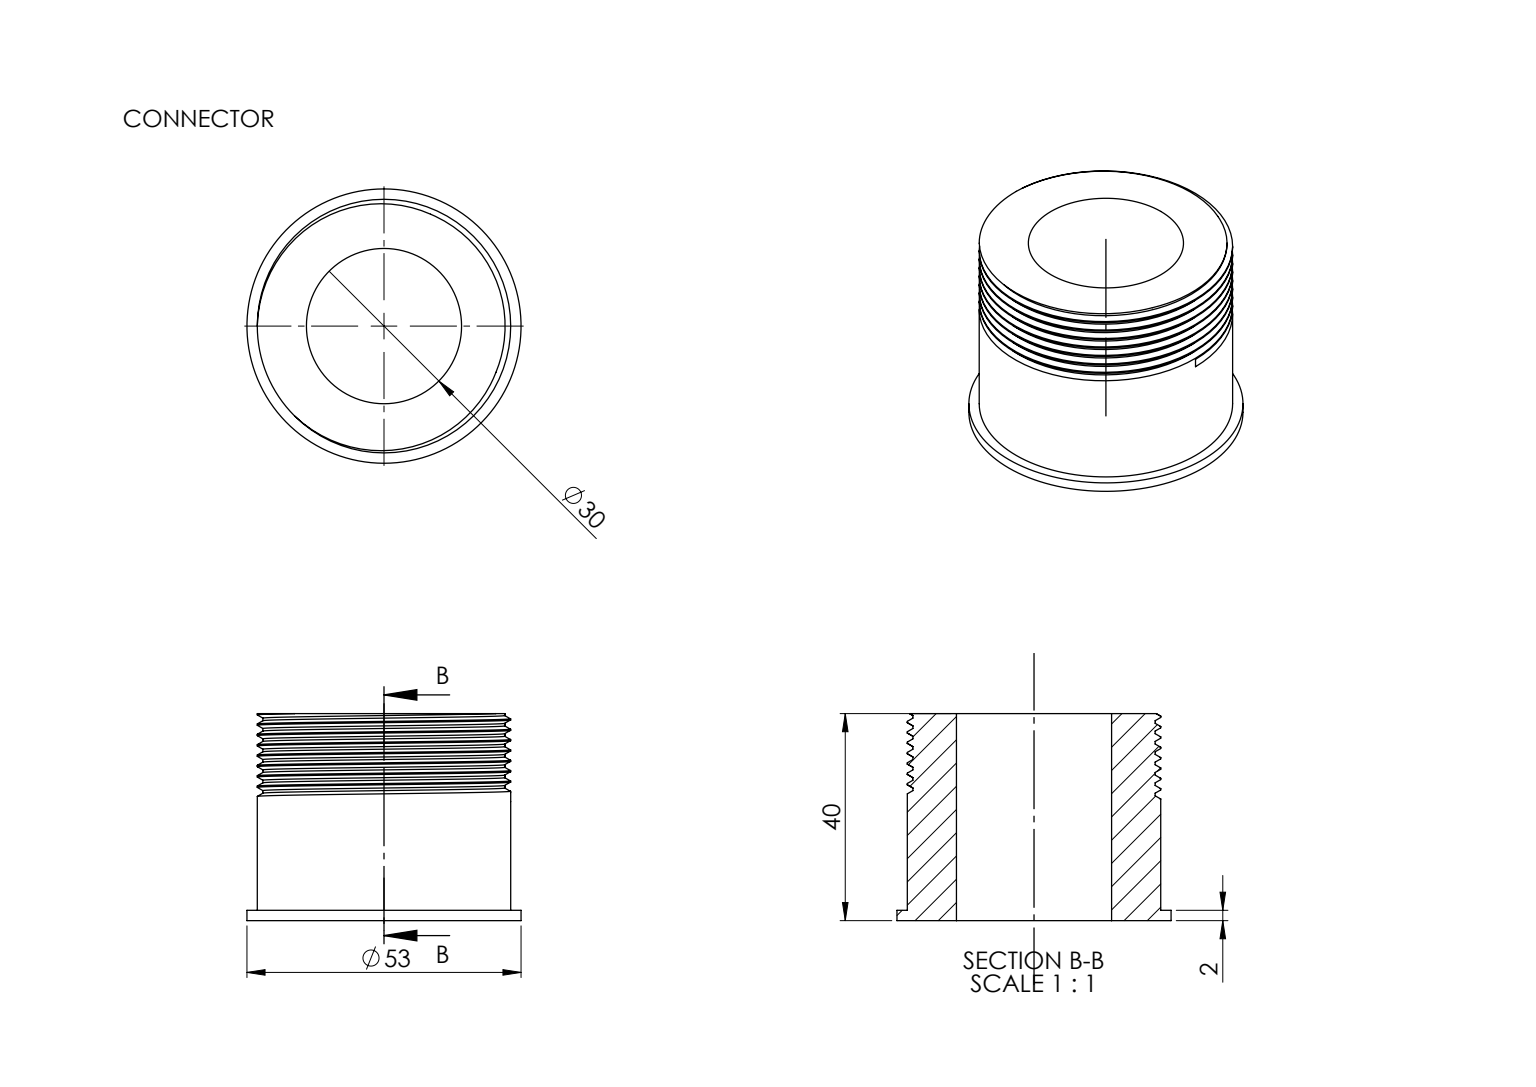
ISO-10303-21;
HEADER;
FILE_DESCRIPTION (('STEP AP214'),
    '1' );
FILE_NAME ('connector.step',
    '2026-10-02T18:08:48',
    ( '' ),
    ( '' ),
    'SwSTEP 2.0',
    'SolidWorks 2026',
    '' );
FILE_SCHEMA (( 'AUTOMOTIVE_DESIGN' ));
ENDSEC;

DATA;
#3=CARTESIAN_POINT ( 'NONE',  ( 7.236395654485760609, 11.52499999726880375, -22.27133577429736633 ) ) ;
#13=CARTESIAN_POINT ( 'NONE',  ( 15.14183272437242067, 5.449999994537614967, 20.84094480462498211 ) ) ;
#22=CARTESIAN_POINT ( 'NONE',  ( 14.47279130897151589, 4.324999997268801799, 19.92008829642072953 ) ) ;
#31=DIRECTION ( 'NONE',  ( 0.000000000000000000, -1.000000000000000000, 0.000000000000000000 ) ) ;
#45=CARTESIAN_POINT ( 'NONE',  ( -14.47279130897151589, 9.324999997268816898, -19.92008829642072598 ) ) ;
#55=EDGE_LOOP ( 'NONE', ( #23841, #28367, #25851, #31674 ) ) ;
#70=CARTESIAN_POINT ( 'NONE',  ( -15.14183272437242600, 17.04999999453762527, 20.84094480462497856 ) ) ;
#86=CARTESIAN_POINT ( 'NONE',  ( -7.236395654485757944, 9.724999997268806595, -22.27133577429736988 ) ) ;
#96=DIRECTION ( 'NONE',  ( 0.000000000000000000, -1.000000000000000000, 0.000000000000000000 ) ) ;
#115=CARTESIAN_POINT ( 'NONE',  ( 0.000000000000000000, 16.99999999999998579, -15.00000000000000000 ) ) ;
#149=CARTESIAN_POINT ( 'NONE',  ( 7.570916362186213000, 8.399999999999991473, -23.30088464923126423 ) ) ;
#161=FACE_OUTER_BOUND ( 'NONE', #7601, .T. ) ;
#173=CARTESIAN_POINT ( 'NONE',  ( -4.523095164977117273E-15, 14.62499999726882649, 24.62258325217400312 ) ) ;
#181=EDGE_CURVE ( 'NONE', #2430, #476, #12819, .T. ) ;
#191=CARTESIAN_POINT ( 'NONE',  ( -7.236395654485763274, 6.024999997268825958, 22.27133577429736633 ) ) ;
#214=CARTESIAN_POINT ( 'NONE',  ( -4.523095164977116484E-15, 12.12499999726881406, 24.62258325217400312 ) ) ;
#242=CARTESIAN_POINT ( 'NONE',  ( 7.236395654485755280, 2.724999997268801266, 22.27133577429736988 ) ) ;
#245=( BOUNDED_CURVE ( )  B_SPLINE_CURVE ( 2, ( #20282, #2248, #31077, #20802, #5337, #28338, #4995 ),
 .UNSPECIFIED., .F., .T. ) 
 B_SPLINE_CURVE_WITH_KNOTS ( ( 3, 2, 2, 3 ),
 ( 0.000000000000000000, 0.01111111111111111154, 0.02222222222222222307, 0.02777777777777777971 ),
 .UNSPECIFIED. ) 
 CURVE ( )  GEOMETRIC_REPRESENTATION_ITEM ( )  RATIONAL_B_SPLINE_CURVE ( ( 1.000000000000000000, 0.9510565162951535312, 1.000000000000000000, 0.9510565162951535312, 1.000000000000000000, 0.9755282581475768211, 0.9755282581475768211 ) ) 
 REPRESENTATION_ITEM ( '' )  );
#257=CARTESIAN_POINT ( 'NONE',  ( -14.47279130897151589, 7.824999997268807128, -19.92008829642072598 ) ) ;
#280=PRODUCT_CONTEXT ( 'NONE', #6136, 'mechanical' ) ;
#294=CARTESIAN_POINT ( 'NONE',  ( 5.270191272235265068, 16.99999999999999645, -22.91526030449972851 ) ) ;
#314=MECHANICAL_DESIGN_GEOMETRIC_PRESENTATION_REPRESENTATION('',(#29900),#24959);
#322=CARTESIAN_POINT ( 'NONE',  ( -7.570916362186215665, 7.399999999999989697, 23.30088464923126423 ) ) ;
#327=CARTESIAN_POINT ( 'NONE',  ( -23.41746824999999887, 1.624999997268811169, -2.867812753649727150E-15 ) ) ;
#328=ADVANCED_FACE ( 'NONE', ( #23862 ), #25917, .T. ) ;
#348=( BOUNDED_CURVE ( )  B_SPLINE_CURVE ( 2, ( #28685, #12736, #2613, #13, #28179, #10501, #4666, #28512, #9994, #20980, #17898, #2090, #20467 ),
 .UNSPECIFIED., .F., .T. ) 
 B_SPLINE_CURVE_WITH_KNOTS ( ( 3, 2, 2, 2, 2, 2, 3 ),
 ( 0.1944444444444444475, 0.2000000000000000111, 0.2111111111111111105, 0.2222222222222222099, 0.2333333333333333370, 0.2444444444444444364, 0.2500000000000000000 ),
 .UNSPECIFIED. ) 
 CURVE ( )  GEOMETRIC_REPRESENTATION_ITEM ( )  RATIONAL_B_SPLINE_CURVE ( ( 0.9755282581475768211, 0.9755282581475768211, 1.000000000000000000, 0.9510565162951535312, 1.000000000000000000, 0.9510565162951535312, 1.000000000000000000, 0.9510565162951535312, 1.000000000000000000, 0.9510565162951535312, 1.000000000000000000, 0.9755282581475767101, 0.9755282581475768211 ) ) 
 REPRESENTATION_ITEM ( '' )  );
#365=CARTESIAN_POINT ( 'NONE',  ( -23.41746825000000243, 7.524999997268816188, -7.608796670333730638 ) ) ;
#375=CARTESIAN_POINT ( 'NONE',  ( 7.236395654485755280, 18.72499999726881370, 22.27133577429736988 ) ) ;
#389=CYLINDRICAL_SURFACE ( 'NONE', #32540, 24.50000000000000000 ) ;
#413=CARTESIAN_POINT ( 'NONE',  ( -18.94512977948576093, 2.324999997268817342, 13.76444248337722698 ) ) ;
#428=CARTESIAN_POINT ( 'NONE',  ( 18.94512977948575738, 14.92499999726881654, 13.76444248337723408 ) ) ;
#430=EDGE_LOOP ( 'NONE', ( #16909, #1055, #4151, #23333 ) ) ;
#441=CARTESIAN_POINT ( 'NONE',  ( -4.223320258572819786E-15, 3.499999999999996891, 24.50000000000000000 ) ) ;
#469=CARTESIAN_POINT ( 'NONE',  ( -24.50000000000000000, 10.74999999453762811, -3.000384657911015469E-15 ) ) ;
#476=VERTEX_POINT ( 'NONE', #13893 ) ;
#492=CARTESIAN_POINT ( 'NONE',  ( -24.50000000000000000, 5.000000000000004441, -3.000384657911015469E-15 ) ) ;
#497=CARTESIAN_POINT ( 'NONE',  ( -23.41746824999999887, 5.624999997268814944, -2.867812753649727150E-15 ) ) ;
#498=CARTESIAN_POINT ( 'NONE',  ( 6.001560367445586717E-15, 3.249999994537631665, 24.50000000000000000 ) ) ;
#505=CYLINDRICAL_SURFACE ( 'NONE', #10621, 24.50000000000000000 ) ;
#515=CARTESIAN_POINT ( 'NONE',  ( -4.523095164977117273E-15, 16.62499999726881583, 24.62258325217400312 ) ) ;
#516=ORIENTED_EDGE ( 'NONE', *, *, #16090, .F. ) ;
#531=CARTESIAN_POINT ( 'NONE',  ( -7.236395654485763274, 8.024999997268828622, 22.27133577429736633 ) ) ;
#539=CARTESIAN_POINT ( 'NONE',  ( 14.47279130897151767, 17.42499999726882365, -19.92008829642072598 ) ) ;
#549=EDGE_CURVE ( 'NONE', #23152, #22342, #16936, .T. ) ;
#554=CARTESIAN_POINT ( 'NONE',  ( 1.507698388325705758E-15, 15.12499999726880873, -24.62258325217400312 ) ) ;
#578=CARTESIAN_POINT ( 'NONE',  ( 24.50000000000000355, 17.84999999453763309, -7.960532557706203605 ) ) ;
#591=CARTESIAN_POINT ( 'NONE',  ( -18.94512977948575738, 11.92499999726881477, -13.76444248337723231 ) ) ;
#594=FACE_OUTER_BOUND ( 'NONE', #26488, .T. ) ;
#609=EDGE_CURVE ( 'NONE', #1393, #3518, #27447, .T. ) ;
#618=EDGE_CURVE ( 'NONE', #4913, #19128, #19343, .T. ) ;
#619=CARTESIAN_POINT ( 'NONE',  ( -19.82091636218621389, 11.19999999999998863, 14.40073868116558842 ) ) ;
#629=CARTESIAN_POINT ( 'NONE',  ( -7.579748464070167083E-14, 12.24999999453762456, -24.50000000000000000 ) ) ;
#658=CARTESIAN_POINT ( 'NONE',  ( 7.570916362186213000, 10.39999999999999325, -23.30088464923126423 ) ) ;
#660=CARTESIAN_POINT ( 'NONE',  ( -15.14183272437241889, 8.449999994537634507, -20.84094480462497856 ) ) ;
#662=CARTESIAN_POINT ( 'NONE',  ( 23.41746824999999887, 10.62499999726881938, 0.000000000000000000 ) ) ;
#666=CARTESIAN_POINT ( 'NONE',  ( 23.41705066890375520, 16.99999999999998934, -0.7769985253002599235 ) ) ;
#683=CARTESIAN_POINT ( 'NONE',  ( 18.94512977948575738, 12.92499999726881654, 13.76444248337723408 ) ) ;
#697=CARTESIAN_POINT ( 'NONE',  ( 7.236395654485755280, 12.22499999726881015, 22.27133577429736988 ) ) ;
#719=CARTESIAN_POINT ( 'NONE',  ( -18.94512977948576093, 15.82499999726880091, 13.76444248337722698 ) ) ;
#744=CARTESIAN_POINT ( 'NONE',  ( -19.82091636218621389, 18.94999999453764161, 14.40073868116558842 ) ) ;
#750=AXIS2_PLACEMENT_3D ( 'NONE', #9964, #23009, #11849 ) ;
#764=CARTESIAN_POINT ( 'NONE',  ( 14.47279130897151767, 15.42499999726879878, -19.92008829642072598 ) ) ;
#795=CARTESIAN_POINT ( 'NONE',  ( -3.331698596277962388, 16.99999999999997868, 23.93330680440991998 ) ) ;
#826=CARTESIAN_POINT ( 'NONE',  ( -24.50000000000000000, 9.000000000000007105, -3.000384657911015469E-15 ) ) ;
#829=CARTESIAN_POINT ( 'NONE',  ( 14.47279130897151767, 12.32499999726880802, 19.92008829642072953 ) ) ;
#844=CARTESIAN_POINT ( 'NONE',  ( -19.82091636218621034, 16.80000000000000782, -14.40073868116559552 ) ) ;
#855=DIRECTION ( 'NONE',  ( 0.000000000000000000, -1.000000000000000000, 0.000000000000000000 ) ) ;
#863=CARTESIAN_POINT ( 'NONE',  ( 18.94512977948575738, 12.42499999726881477, 13.76444248337723408 ) ) ;
#885=CARTESIAN_POINT ( 'NONE',  ( 7.236395654485760609, 13.02499999726880375, -22.27133577429736633 ) ) ;
#890=CARTESIAN_POINT ( 'NONE',  ( -14.47279130897152299, 4.424999997268826313, 19.92008829642072243 ) ) ;
#910=ORIENTED_EDGE ( 'NONE', *, *, #33041, .T. ) ;
#911=CARTESIAN_POINT ( 'NONE',  ( 7.236395654485760609, 9.524999997268828622, -22.27133577429736633 ) ) ;
#926=CARTESIAN_POINT ( 'NONE',  ( -7.236395654485763274, 14.52499999726880553, 22.27133577429736633 ) ) ;
#935=CARTESIAN_POINT ( 'NONE',  ( -3.880418787951137816, 0.5512542815468468582, -24.49999999999999645 ) ) ;
#956=CARTESIAN_POINT ( 'NONE',  ( -6.700584085799521361, 16.99999999999998934, 23.28199799329060582 ) ) ;
#963=CARTESIAN_POINT ( 'NONE',  ( -3.880418787951156023, 10.30125427608447453, -24.49999999999999645 ) ) ;
#975=CARTESIAN_POINT ( 'NONE',  ( 24.50000000000000000, 15.84999999453763664, -7.960532557706203605 ) ) ;
#986=CARTESIAN_POINT ( 'NONE',  ( -24.50000000000000355, 14.89999999999999680, -7.960532557706207157 ) ) ;
#990=CARTESIAN_POINT ( 'NONE',  ( -7.236395654485763274, 10.02499999726880198, 22.27133577429736633 ) ) ;
#991=CARTESIAN_POINT ( 'NONE',  ( -1.756012107511856980E-14, 4.499999999999997335, -24.50000000000000000 ) ) ;
#994=CARTESIAN_POINT ( 'NONE',  ( 19.05376897654620194, 16.99999999999997868, -13.63518129362208953 ) ) ;
#1023=CARTESIAN_POINT ( 'NONE',  ( 18.94512977948576093, 12.82499999726882578, -13.76444248337722875 ) ) ;
#1049=CARTESIAN_POINT ( 'NONE',  ( -23.41746825000000243, 4.224999997268803931, 7.608796670333725309 ) ) ;
#1055=ORIENTED_EDGE ( 'NONE', *, *, #4319, .F. ) ;
#1072=CARTESIAN_POINT ( 'NONE',  ( -14.47279130897151589, 7.824999997268807128, -19.92008829642072598 ) ) ;
#1082=CARTESIAN_POINT ( 'NONE',  ( -7.579748464070165821E-14, 16.50000000000000355, -24.50000000000000000 ) ) ;
#1087=CARTESIAN_POINT ( 'NONE',  ( 23.41746825000000243, 17.22499999726880304, -7.608796670333727974 ) ) ;
#1095=CARTESIAN_POINT ( 'NONE',  ( -24.50000000000000000, 0.9000000000000005773, -7.960532557706207157 ) ) ;
#1096=EDGE_LOOP ( 'NONE', ( #14624, #31167 ) ) ;
#1109=CARTESIAN_POINT ( 'NONE',  ( -15.14183272437242067, 16.44999999453761674, -20.84094480462497856 ) ) ;
#1110=CARTESIAN_POINT ( 'NONE',  ( 7.313012447739250820E-14, 15.50000000000000178, 24.50000000000000000 ) ) ;
#1116=CARTESIAN_POINT ( 'NONE',  ( 20.86390607985937606, 16.99999999999997868, 10.74782858706267952 ) ) ;
#1153=CARTESIAN_POINT ( 'NONE',  ( 24.50000000000000000, 12.00000000000001066, 0.000000000000000000 ) ) ;
#1157=CARTESIAN_POINT ( 'NONE',  ( -14.47279130897152299, 11.92499999726882187, 19.92008829642072243 ) ) ;
#1159=CARTESIAN_POINT ( 'NONE',  ( 19.82091636218621389, 3.949999994537628289, -14.40073868116559197 ) ) ;
#1193=CARTESIAN_POINT ( 'NONE',  ( -4.523095164977116484E-15, 10.12499999726881938, 24.62258325217400312 ) ) ;
#1199=ORIENTED_EDGE ( 'NONE', *, *, #16507, .F. ) ;
#1229=CARTESIAN_POINT ( 'NONE',  ( -1.756012107511856980E-14, 4.499999999999997335, -24.50000000000000000 ) ) ;
#1232=( BOUNDED_CURVE ( )  B_SPLINE_CURVE ( 2, ( #19854, #17980, #28430, #1483, #30308, #11957, #32875, #6807, #9374, #17286, #27749, #14711, #441 ),
 .UNSPECIFIED., .F., .T. ) 
 B_SPLINE_CURVE_WITH_KNOTS ( ( 3, 2, 2, 2, 2, 2, 3 ),
 ( 0.1388888888888888951, 0.1444444444444444309, 0.1555555555555555580, 0.1666666666666666574, 0.1777777777777777846, 0.1888888888888888840, 0.1944444444444444475 ),
 .UNSPECIFIED. ) 
 CURVE ( )  GEOMETRIC_REPRESENTATION_ITEM ( )  RATIONAL_B_SPLINE_CURVE ( ( 0.9755282581475768211, 0.9755282581475768211, 1.000000000000000000, 0.9510565162951535312, 1.000000000000000000, 0.9510565162951535312, 1.000000000000000000, 0.9510565162951535312, 1.000000000000000000, 0.9510565162951535312, 1.000000000000000000, 0.9755282581475768211, 0.9755282581475768211 ) ) 
 REPRESENTATION_ITEM ( '' )  );
#1241=CARTESIAN_POINT ( 'NONE',  ( -23.41746825000000598, 4.224999997268803931, 7.608796670333726198 ) ) ;
#1255=CARTESIAN_POINT ( 'NONE',  ( -4.523095164977116484E-15, 18.62499999726881583, 24.62258325217400312 ) ) ;
#1263=ORIENTED_EDGE ( 'NONE', *, *, #19113, .T. ) ;
#1281=CARTESIAN_POINT ( 'NONE',  ( 19.82091636218621034, 9.549999994537621717, 14.40073868116559730 ) ) ;
#1295=CARTESIAN_POINT ( 'NONE',  ( 23.41746825000000243, 3.024999997268812635, 7.608796670333735079 ) ) ;
#1324=CARTESIAN_POINT ( 'NONE',  ( 19.82091636218621034, 9.800000000000002487, 14.40073868116559730 ) ) ;
#1329=CARTESIAN_POINT ( 'NONE',  ( 23.41746824999999887, 12.52499999726880375, 7.608796670333735079 ) ) ;
#1334=CARTESIAN_POINT ( 'NONE',  ( -7.570916362186215665, 5.149999994537635573, 23.30088464923126423 ) ) ;
#1335=DIRECTION ( 'NONE',  ( -0.8660254037844399289, -0.4999999999999977240, 0.000000000000000000 ) ) ;
#1366=CARTESIAN_POINT ( 'NONE',  ( 23.41746825000000243, 10.72499999726880127, -7.608796670333727974 ) ) ;
#1373=EDGE_CURVE ( 'NONE', #11531, #13996, #14522, .T. ) ;
#1376=AXIS2_PLACEMENT_3D ( 'NONE', #6186, #27460, #21818 ) ;
#1378=CARTESIAN_POINT ( 'NONE',  ( 3.000384657911015469E-15, 16.99999999999998579, 24.50000000000000000 ) ) ;
#1393=VERTEX_POINT ( 'NONE', #7954 ) ;
#1409=SURFACE_SIDE_STYLE ('',( #16544 ) ) ;
#1416=CARTESIAN_POINT ( 'NONE',  ( 23.41746825000000243, 9.024999997268826846, 7.608796670333735079 ) ) ;
#1427=CARTESIAN_POINT ( 'NONE',  ( 7.570916362186207671, 7.349999994537615322, 23.30088464923126779 ) ) ;
#1429=CARTESIAN_POINT ( 'NONE',  ( 23.41746825000000243, 4.724999997268818142, -7.608796670333727974 ) ) ;
#1454=CARTESIAN_POINT ( 'NONE',  ( -19.82091636218621034, 4.549999994537618164, -14.40073868116559552 ) ) ;
#1463=ADVANCED_FACE ( 'NONE', ( #2982 ), #389, .T. ) ;
#1471=CARTESIAN_POINT ( 'NONE',  ( 14.47279130897151589, 2.824999997268819119, 19.92008829642072953 ) ) ;
#1483=CARTESIAN_POINT ( 'NONE',  ( -15.14183272437242067, 2.700000000000001954, -20.84094480462497856 ) ) ;
#1497=CARTESIAN_POINT ( 'NONE',  ( -15.14183272437241889, 16.69999999999999574, -20.84094480462497856 ) ) ;
#1501=CARTESIAN_POINT ( 'NONE',  ( 23.41746824999999887, 16.62499999726882294, 0.000000000000000000 ) ) ;
#1536=CARTESIAN_POINT ( 'NONE',  ( 14.47279130897151767, 14.92499999726881299, -19.92008829642072598 ) ) ;
#1558=CARTESIAN_POINT ( 'NONE',  ( 23.41746824999999887, 3.124999997268812280, 0.000000000000000000 ) ) ;
#1575=DIRECTION ( 'NONE',  ( 0.000000000000000000, -1.000000000000000000, 0.000000000000000000 ) ) ;
#1582=CARTESIAN_POINT ( 'NONE',  ( -18.94512977948576093, 4.324999997268818674, 13.76444248337722698 ) ) ;
#1594=CARTESIAN_POINT ( 'NONE',  ( -14.47279130897152122, 5.924999997268808549, 19.92008829642072243 ) ) ;
#1618=CARTESIAN_POINT ( 'NONE',  ( 1.555960095263670572E-15, 14.24999999453762278, -24.50000000000000000 ) ) ;
#1620=CARTESIAN_POINT ( 'NONE',  ( 7.570916362186213000, 4.149999994537633796, -23.30088464923126423 ) ) ;
#1634=CARTESIAN_POINT ( 'NONE',  ( -14.47279130897152122, 2.424999997268802332, 19.92008829642072243 ) ) ;
#1648=CARTESIAN_POINT ( 'NONE',  ( 1.555960095263670572E-15, 8.249999994537619230, -24.50000000000000000 ) ) ;
#1669=CARTESIAN_POINT ( 'NONE',  ( 18.94512977948576093, 14.82499999726880091, -13.76444248337722875 ) ) ;
#1673=CARTESIAN_POINT ( 'NONE',  ( -4.223320258572819786E-15, 5.249999994537629888, 24.50000000000000000 ) ) ;
#1704=CARTESIAN_POINT ( 'NONE',  ( 24.50000000000000355, 0.09999999999999684142, -7.960532557706203605 ) ) ;
#1728=CARTESIAN_POINT ( 'NONE',  ( -7.236395654485757944, 5.724999997268803931, -22.27133577429736988 ) ) ;
#1748=CARTESIAN_POINT ( 'NONE',  ( 19.82091636218621389, 8.200000000000013500, -14.40073868116559197 ) ) ;
#1751=ORIENTED_EDGE ( 'NONE', *, *, #28129, .T. ) ;
#1752=CARTESIAN_POINT ( 'NONE',  ( 23.41746824999999887, 13.12499999726882116, 0.000000000000000000 ) ) ;
#1753=CARTESIAN_POINT ( 'NONE',  ( 23.41746824999999887, 0.6249999972688102812, 0.000000000000000000 ) ) ;
#1765=CARTESIAN_POINT ( 'NONE',  ( 18.94512977948576093, 0.8249999972688160099, -13.76444248337722875 ) ) ;
#1793=CARTESIAN_POINT ( 'NONE',  ( -4.732186688966233175E-15, 7.249999994537616566, 25.76082449383753925 ) ) ;
#1809=CARTESIAN_POINT ( 'NONE',  ( -7.236395654485757944, 3.724999997268802154, -22.27133577429736988 ) ) ;
#1844=FACE_OUTER_BOUND ( 'NONE', #14245, .T. ) ;
#1875=CARTESIAN_POINT ( 'NONE',  ( 24.50000000000000000, 13.64999999453761781, 7.960532557706212486 ) ) ;
#1880=CARTESIAN_POINT ( 'NONE',  ( -15.14183272437241889, 0.7000000000000070610, -20.84094480462497856 ) ) ;
#1882=DIRECTION ( 'NONE',  ( 0.000000000000000000, -0.000000000000000000, -1.000000000000000000 ) ) ;
#1907=CARTESIAN_POINT ( 'NONE',  ( 14.47279130897151767, 8.824999997268804464, 19.92008829642072953 ) ) ;
#1927=CARTESIAN_POINT ( 'NONE',  ( 7.570916362186213000, 8.399999999999991473, -23.30088464923126423 ) ) ;
#1931=CARTESIAN_POINT ( 'NONE',  ( 18.94512977948576093, 15.32499999726880091, -13.76444248337722875 ) ) ;
#1932=CARTESIAN_POINT ( 'NONE',  ( 14.47279130897151944, 0.9249999972688209837, -19.92008829642072598 ) ) ;
#1947=CARTESIAN_POINT ( 'NONE',  ( -23.41746825000000243, 3.524999997268826402, -7.608796670333730638 ) ) ;
#1949=STYLED_ITEM ( 'NONE', ( #25225 ), #13626 ) ;
#1952=( BOUNDED_CURVE ( )  B_SPLINE_CURVE ( 2, ( #2358, #18503, #16757, #1109, #19331, #11594, #27216, #6281, #3378, #3709, #14179 ),
 .UNSPECIFIED., .F., .T. ) 
 B_SPLINE_CURVE_WITH_KNOTS ( ( 3, 2, 2, 2, 2, 3 ),
 ( 0.8055555555555555802, 0.8111111111111111160, 0.8222222222222221877, 0.8333333333333333703, 0.8444444444444444420, 0.8472738309268738055 ),
 .UNSPECIFIED. ) 
 CURVE ( )  GEOMETRIC_REPRESENTATION_ITEM ( )  RATIONAL_B_SPLINE_CURVE ( ( 0.9755282581475768211, 0.9755282581475768211, 1.000000000000000000, 0.9510565162951535312, 1.000000000000000000, 0.9510565162951535312, 1.000000000000000000, 0.9510565162951535312, 1.000000000000000000, 0.9875367971922254240, 0.9814209735438276239 ) ) 
 REPRESENTATION_ITEM ( '' )  );
#1961=VECTOR ( 'NONE', #29560, 1000.000000000000000 ) ;
#1974=CARTESIAN_POINT ( 'NONE',  ( 15.14183272437241889, 15.44999999453761852, 20.84094480462498211 ) ) ;
#1987=CARTESIAN_POINT ( 'NONE',  ( -14.47279130897151589, 1.824999997268821339, -19.92008829642072598 ) ) ;
#1993=ORIENTED_EDGE ( 'NONE', *, *, #6515, .F. ) ;
#2021=CARTESIAN_POINT ( 'NONE',  ( 23.41746824999999887, 14.62499999726882294, 0.000000000000000000 ) ) ;
#2022=VECTOR ( 'NONE', #3479, 1000.000000000000000 ) ;
#2026=CARTESIAN_POINT ( 'NONE',  ( -24.50000000000000711, 4.849999994537633974, 7.960532557706201828 ) ) ;
#2038=ORIENTED_EDGE ( 'NONE', *, *, #18277, .T. ) ;
#2056=CARTESIAN_POINT ( 'NONE',  ( 23.41746825000000243, 16.72499999726881725, -7.608796670333727974 ) ) ;
#2062=ORIENTED_EDGE ( 'NONE', *, *, #16915, .F. ) ;
#2071=CARTESIAN_POINT ( 'NONE',  ( 7.570916362186207671, 5.599999999999994316, 23.30088464923126779 ) ) ;
#2075=CARTESIAN_POINT ( 'NONE',  ( 19.82091636218621034, 7.549999994537620829, 14.40073868116559730 ) ) ;
#2082=CARTESIAN_POINT ( 'NONE',  ( -23.41746824999999887, 8.024999997268800200, -7.608796670333730638 ) ) ;
#2090=CARTESIAN_POINT ( 'NONE',  ( 3.880418787951132042, 6.198745712990783474, -24.50000000000000355 ) ) ;
#2098=CARTESIAN_POINT ( 'NONE',  ( -18.94512977948575738, 1.424999997268805441, -13.76444248337723231 ) ) ;
#2107=CARTESIAN_POINT ( 'NONE',  ( 14.47279130897151589, 14.82499999726881690, 19.92008829642072953 ) ) ;
#2108=CARTESIAN_POINT ( 'NONE',  ( 18.94512977948575738, 4.424999997268807661, 13.76444248337723408 ) ) ;
#2120=CARTESIAN_POINT ( 'NONE',  ( -23.41746825000000243, 9.524999997268810858, -7.608796670333730638 ) ) ;
#2143=CARTESIAN_POINT ( 'NONE',  ( 19.82091636218621034, 15.54999999453762705, 14.40073868116559730 ) ) ;
#2157=CARTESIAN_POINT ( 'NONE',  ( 14.47279130897151589, 10.82499999726882756, 19.92008829642072953 ) ) ;
#2184=CARTESIAN_POINT ( 'NONE',  ( -24.50000000000000000, 16.99999999999998579, -3.000384657911015469E-15 ) ) ;
#2189=CARTESIAN_POINT ( 'NONE',  ( -7.236395654485763274, 16.02499999726880731, 22.27133577429736633 ) ) ;
#2206=DIRECTION ( 'NONE',  ( 0.000000000000000000, -1.000000000000000000, 0.000000000000000000 ) ) ;
#2220=( NAMED_UNIT ( * ) PLANE_ANGLE_UNIT ( ) SI_UNIT ( $, .RADIAN. ) );
#2224=CARTESIAN_POINT ( 'NONE',  ( 23.41746825000000243, 16.52499999726882152, 7.608796670333735079 ) ) ;
#2248=CARTESIAN_POINT ( 'NONE',  ( 24.50000000000000000, 0.09999999999999682754, -7.960532557706203605 ) ) ;
#2253=CARTESIAN_POINT ( 'NONE',  ( 14.47279130897151944, 7.424999997268819207, -19.92008829642072598 ) ) ;
#2271=CARTESIAN_POINT ( 'NONE',  ( 18.94512977948576093, 0.8249999972688160099, -13.76444248337722875 ) ) ;
#2280=CARTESIAN_POINT ( 'NONE',  ( 23.41746824999999887, 11.12499999726881938, 0.000000000000000000 ) ) ;
#2281=CARTESIAN_POINT ( 'NONE',  ( 18.94512977948576093, 4.824999997268819563, -13.76444248337722875 ) ) ;
#2296=CARTESIAN_POINT ( 'NONE',  ( -14.47279130897151589, 11.32499999726881157, -19.92008829642072598 ) ) ;
#2298=ORIENTED_EDGE ( 'NONE', *, *, #30160, .T. ) ;
#2319=CARTESIAN_POINT ( 'NONE',  ( -15.14183272437242600, 13.04999999453763770, 20.84094480462497856 ) ) ;
#2333=AXIS2_PLACEMENT_3D ( 'NONE', #21565, #16419, #19157 ) ;
#2334=CARTESIAN_POINT ( 'NONE',  ( -7.236395654485757944, 5.724999997268803931, -22.27133577429736988 ) ) ;
#2339=ORIENTED_EDGE ( 'NONE', *, *, #18402, .F. ) ;
#2358=CARTESIAN_POINT ( 'NONE',  ( 1.555960095263670572E-15, 16.24999999453762101, -24.50000000000000000 ) ) ;
#2368=B_SPLINE_CURVE_WITH_KNOTS ( 'NONE', 3,
 ( #13729, #11643, #22127, #32240, #9070, #31901, #19550, #16976, #29653, #32403, #8396, #16642, #994, #6333, #18883, #11479, #13569, #5833, #16471, #3259, #24196, #29491, #666, #5995, #12148, #30852, #4260, #25546, #32737, #25195, #27947, #25025 ),
 .UNSPECIFIED., .F., .F.,
 ( 4, 2, 2, 2, 2, 2, 2, 2, 2, 2, 2, 2, 2, 2, 2, 4 ),
 ( 0.000000000000000000, 0.002298871809599534188, 0.004597743619199068377, 0.006896615428798602565, 0.009195487238398136753, 0.01149435904799767094, 0.01379323085759720513, 0.01609210266719673932, 0.01839097447679627351, 0.02298871809599534188, 0.02528758990559487607, 0.02758646171519441026, 0.02988533352479394445, 0.03218420533439347864, 0.03448307714399301283, 0.03678194895359254701 ),
 .UNSPECIFIED. ) ;
#2396=EDGE_CURVE ( 'NONE', #3518, #19128, #27625, .T. ) ;
#2405=CARTESIAN_POINT ( 'NONE',  ( 15.14183272437241889, 5.699999999999993960, 20.84094480462498211 ) ) ;
#2411=VECTOR ( 'NONE', #14860, 1000.000000000000000 ) ;
#2417=PLANE ( 'NONE',  #7272 ) ;
#2429=CARTESIAN_POINT ( 'NONE',  ( 23.41746824999999887, 9.024999997268826846, 7.608796670333735079 ) ) ;
#2430=VERTEX_POINT ( 'NONE', #11664 ) ;
#2438=FACE_OUTER_BOUND ( 'NONE', #21729, .T. ) ;
#2456=CARTESIAN_POINT ( 'NONE',  ( -23.41746825000000598, 12.22499999726881370, 7.608796670333726198 ) ) ;
#2457=CARTESIAN_POINT ( 'NONE',  ( 14.47279130897151944, 2.924999997268816099, -19.92008829642072598 ) ) ;
#2469=CARTESIAN_POINT ( 'NONE',  ( 7.236395654485760609, 7.024999997268826846, -22.27133577429736633 ) ) ;
#2471=DIRECTION ( 'NONE',  ( 0.000000000000000000, 0.000000000000000000, -1.000000000000000000 ) ) ;
#2494=CARTESIAN_POINT ( 'NONE',  ( 7.570916362186213000, 14.14999999453761603, -23.30088464923126423 ) ) ;
#2510=CARTESIAN_POINT ( 'NONE',  ( -18.94512977948575738, 5.924999997268809437, -13.76444248337723231 ) ) ;
#2519=ORIENTED_EDGE ( 'NONE', *, *, #7482, .F. ) ;
#2521=CARTESIAN_POINT ( 'NONE',  ( 3.880418787951102289, 10.44874571845314470, -24.50000000000000711 ) ) ;
#2529=CARTESIAN_POINT ( 'NONE',  ( -19.82091636218621034, 4.799999999999998934, -14.40073868116559552 ) ) ;
#2542=AXIS2_PLACEMENT_3D ( 'NONE', #19089, #31, #24235 ) ;
#2581=CARTESIAN_POINT ( 'NONE',  ( -24.50000000000000355, 2.899999999999995470, -7.960532557706207157 ) ) ;
#2586=DIRECTION ( 'NONE',  ( 0.000000000000000000, -1.000000000000000000, 0.000000000000000000 ) ) ;
#2590=LINE ( 'NONE', #28030, #25348 ) ;
#2605=CARTESIAN_POINT ( 'NONE',  ( -14.47279130897152299, 12.42499999726880588, 19.92008829642072243 ) ) ;
#2613=CARTESIAN_POINT ( 'NONE',  ( 7.570916362186207671, 5.349999994537641079, 23.30088464923126779 ) ) ;
#2621=CARTESIAN_POINT ( 'NONE',  ( -18.94512977948576093, 5.824999997268820451, 13.76444248337722698 ) ) ;
#2643=CARTESIAN_POINT ( 'NONE',  ( -14.47279130897152122, 9.924999997268825425, 19.92008829642072243 ) ) ;
#2658=CARTESIAN_POINT ( 'NONE',  ( -19.82091636218621034, 6.549999994537619941, -14.40073868116559552 ) ) ;
#2670=CARTESIAN_POINT ( 'NONE',  ( -7.570916362186210335, 10.34999999453761710, -23.30088464923126779 ) ) ;
#2673=( BOUNDED_SURFACE ( )  B_SPLINE_SURFACE ( 1, 2, ( 
 ( #20020, #12111, #9194, #25331, #15043, #33034, #9887, #1987, #19679, #24988, #20364, #27566, #12462, #1634, #22932, #9712, #33388, #1471, #7134, #1295, #25157, #4393, #30812, #22583, #7305, #30125, #1809, #11777, #6795, #6628, #22257, #9538, #17789, #17107, #4053, #11946, #22415, #6965, #32863, #9360, #12285, #22759, #19841, #33210, #12977, #15388, #2334, #18311, #2510, #18478, #23279, #2685, #10574, #33565, #4907, #31664, #10403, #28922, #28583, #8159, #33914, #20882, #7994, #13144, #21221, #31331, #26190, #257, #7823, #28757, #5253, #18649, #29087, #5422, #31501, #15735, #10063, #15902, #18139, #12807, #10239, #23617, #28418, #21052, #15213, #13318, #86, #17968, #23452, #26357, #31161, #2847, #25676, #10742, #25844, #23791, #5080, #2157, #26018, #12631, #23101, #20543, #30988, #7488, #33744, #20720, #15566, #7653, #591, #29425, #22049, #5927, #16404, #18813, #29256, #6256, #3683, #29582, #5759, #8824, #16735, #13824, #19309, #26528, #29751, #27192, #18980, #13988, #3021, #24293, #3354, #24450, #13492, #11245, #926, #19475, #8493, #8660, #428, #5591, #24125, #16073, #21722, #764, #32496, #26859, #14156, #10913, #32167, #6085, #26694, #23957, #11405, #16239, #19144, #24613, #16567, #27022, #3517, #21882, #32332, #1087, #11569, #8995, #11082, #21385, #31830, #8323, #3190, #13661, #31997, #21551, #33171, #4525, #27526, #1255, #9675, #17067, #4015, #27871, #14489 ),
 ( #25295, #9499, #1765, #17409, #30426, #24947, #6925, #4353, #12072, #14829, #22723, #12246, #14322, #25119, #17236, #3847, #19980, #20155, #4187, #15001, #30600, #24777, #30084, #25470, #32663, #7095, #6757, #17579, #28039, #1947, #19641, #12423, #33350, #9318, #32991, #22893, #22379, #9848, #11736, #29925, #6427, #1429, #22216, #16900, #19805, #27362, #9158, #6590, #11907, #32827, #30253, #27696, #14659, #1594, #22542, #31288, #13106, #4870, #25977, #23064, #28884, #17931, #4696, #10027, #2469, #12935, #15350, #7446, #31122, #5382, #20682, #25641, #12593, #18268, #23411, #33701, #10202, #10365, #18440, #33524, #7265, #30775, #18095, #23579, #10533, #20843, #15861, #45, #33872, #2120, #15524, #28381, #7782, #2643, #17751, #28716, #7615, #25804, #28542, #21010, #5212, #31460, #20325, #20501, #26147, #15695, #7953, #2296, #12768, #26317, #2806, #13273, #30949, #23748, #23242, #214, #28210, #15176, #5039, #24086, #16200, #18941, #11367, #11205, #885, #10700, #10873, #16523, #32124, #24248, #26654, #5722, #21843, #13621, #3149, #21348, #13946, #19265, #8280, #16031, #24409, #31789, #18772, #8620, #29216, #554, #11040, #32288, #29386, #21508, #8781, #6042, #719, #26975, #19102, #21676, #31957, #29540, #3475, #26818, #29707, #6210, #16691, #29047, #5886, #8450, #18608, #27148, #3641, #16363, #14115, #24573, #5550, #3314, #21181, #13449, #31623, #13780, #8121, #26486, #2981 ) ),
 .UNSPECIFIED., .F., .F., .T. ) 
 B_SPLINE_SURFACE_WITH_KNOTS ( ( 2, 2 ),
 ( 3, 2, 2, 2, 2, 2, 2, 2, 2, 2, 2, 2, 2, 2, 2, 2, 2, 2, 2, 2, 2, 2, 2, 2, 2, 2, 2, 2, 2, 2, 2, 2, 2, 2, 2, 2, 2, 2, 2, 2, 2, 2, 2, 2, 2, 2, 2, 2, 2, 2, 2, 2, 2, 2, 2, 2, 2, 2, 2, 2, 2, 2, 2, 2, 2, 2, 2, 2, 2, 2, 2, 2, 2, 2, 2, 2, 2, 2, 2, 2, 2, 2, 2, 2, 2, 2, 2, 2, 2, 2, 3 ),
 ( 0.000000000000000000, 1.000000000000000000 ),
 ( 0.000000000000000000, 0.01111111111111111154, 0.02222222222222222307, 0.03333333333333333287, 0.04444444444444444614, 0.05555555555555555247, 0.06666666666666666574, 0.07777777777777777901, 0.08888888888888889228, 0.1000000000000000056, 0.1111111111111111049, 0.1222222222222222182, 0.1333333333333333315, 0.1444444444444444309, 0.1555555555555555580, 0.1666666666666666574, 0.1777777777777777846, 0.1888888888888888840, 0.2000000000000000111, 0.2111111111111111105, 0.2222222222222222099, 0.2333333333333333370, 0.2444444444444444364, 0.2555555555555555358, 0.2666666666666666630, 0.2777777777777777901, 0.2888888888888888618, 0.2999999999999999889, 0.3111111111111111160, 0.3222222222222222432, 0.3333333333333333148, 0.3444444444444444420, 0.3555555555555555691, 0.3666666666666666408, 0.3777777777777777679, 0.3888888888888888951, 0.4000000000000000222, 0.4111111111111110938, 0.4222222222222222210, 0.4333333333333333481, 0.4444444444444444198, 0.4555555555555555469, 0.4666666666666666741, 0.4777777777777778012, 0.4888888888888888729, 0.5000000000000000000, 0.5111111111111110716, 0.5222222222222222543, 0.5333333333333333259, 0.5444444444444443976, 0.5555555555555555802, 0.5666666666666666519, 0.5777777777777777235, 0.5888888888888889062, 0.5999999999999999778, 0.6111111111111111605, 0.6222222222222222321, 0.6333333333333333037, 0.6444444444444444864, 0.6555555555555555580, 0.6666666666666666297, 0.6777777777777778123, 0.6888888888888888840, 0.6999999999999999556, 0.7111111111111111382, 0.7222222222222222099, 0.7333333333333332815, 0.7444444444444444642, 0.7555555555555555358, 0.7666666666666667185, 0.7777777777777777901, 0.7888888888888888618, 0.8000000000000000444, 0.8111111111111111160, 0.8222222222222221877, 0.8333333333333333703, 0.8444444444444444420, 0.8555555555555555136, 0.8666666666666666963, 0.8777777777777777679, 0.8888888888888888395, 0.9000000000000000222, 0.9111111111111110938, 0.9222222222222222765, 0.9333333333333333481, 0.9444444444444444198, 0.9555555555555556024, 0.9666666666666666741, 0.9777777777777777457, 0.9888888888888889284, 1.000000000000000000 ),
 .UNSPECIFIED. ) 
 GEOMETRIC_REPRESENTATION_ITEM ( )  RATIONAL_B_SPLINE_SURFACE ( (
 ( 1.000000000000000000, 0.9510565162951535312, 1.000000000000000000, 0.9510565162951535312, 1.000000000000000000, 0.9510565162951535312, 1.000000000000000000, 0.9510565162951535312, 1.000000000000000000, 0.9510565162951535312, 1.000000000000000000, 0.9510565162951535312, 1.000000000000000000, 0.9510565162951535312, 1.000000000000000000, 0.9510565162951535312, 1.000000000000000000, 0.9510565162951535312, 1.000000000000000000, 0.9510565162951535312, 1.000000000000000000, 0.9510565162951535312, 1.000000000000000000, 0.9510565162951535312, 1.000000000000000000, 0.9510565162951535312, 1.000000000000000000, 0.9510565162951535312, 1.000000000000000000, 0.9510565162951535312, 1.000000000000000000, 0.9510565162951535312, 1.000000000000000000, 0.9510565162951535312, 1.000000000000000000, 0.9510565162951535312, 1.000000000000000000, 0.9510565162951535312, 1.000000000000000000, 0.9510565162951535312, 1.000000000000000000, 0.9510565162951535312, 1.000000000000000000, 0.9510565162951535312, 1.000000000000000000, 0.9510565162951535312, 1.000000000000000000, 0.9510565162951535312, 1.000000000000000000, 0.9510565162951535312, 1.000000000000000000, 0.9510565162951535312, 1.000000000000000000, 0.9510565162951535312, 1.000000000000000000, 0.9510565162951535312, 1.000000000000000000, 0.9510565162951535312, 1.000000000000000000, 0.9510565162951535312, 1.000000000000000000, 0.9510565162951535312, 1.000000000000000000, 0.9510565162951535312, 1.000000000000000000, 0.9510565162951535312, 1.000000000000000000, 0.9510565162951535312, 1.000000000000000000, 0.9510565162951535312, 1.000000000000000000, 0.9510565162951535312, 1.000000000000000000, 0.9510565162951535312, 1.000000000000000000, 0.9510565162951535312, 1.000000000000000000, 0.9510565162951535312, 1.000000000000000000, 0.9510565162951535312, 1.000000000000000000, 0.9510565162951535312, 1.000000000000000000, 0.9510565162951535312, 1.000000000000000000, 0.9510565162951535312, 1.000000000000000000, 0.9510565162951535312, 1.000000000000000000, 0.9510565162951535312, 1.000000000000000000, 0.9510565162951535312, 1.000000000000000000, 0.9510565162951535312, 1.000000000000000000, 0.9510565162951535312, 1.000000000000000000, 0.9510565162951535312, 1.000000000000000000, 0.9510565162951535312, 1.000000000000000000, 0.9510565162951535312, 1.000000000000000000, 0.9510565162951535312, 1.000000000000000000, 0.9510565162951535312, 1.000000000000000000, 0.9510565162951535312, 1.000000000000000000, 0.9510565162951535312, 1.000000000000000000, 0.9510565162951535312, 1.000000000000000000, 0.9510565162951535312, 1.000000000000000000, 0.9510565162951535312, 1.000000000000000000, 0.9510565162951535312, 1.000000000000000000, 0.9510565162951535312, 1.000000000000000000, 0.9510565162951535312, 1.000000000000000000, 0.9510565162951535312, 1.000000000000000000, 0.9510565162951535312, 1.000000000000000000, 0.9510565162951535312, 1.000000000000000000, 0.9510565162951535312, 1.000000000000000000, 0.9510565162951535312, 1.000000000000000000, 0.9510565162951535312, 1.000000000000000000, 0.9510565162951535312, 1.000000000000000000, 0.9510565162951535312, 1.000000000000000000, 0.9510565162951535312, 1.000000000000000000, 0.9510565162951535312, 1.000000000000000000, 0.9510565162951535312, 1.000000000000000000, 0.9510565162951535312, 1.000000000000000000, 0.9510565162951535312, 1.000000000000000000, 0.9510565162951535312, 1.000000000000000000, 0.9510565162951535312, 1.000000000000000000, 0.9510565162951535312, 1.000000000000000000, 0.9510565162951535312, 1.000000000000000000, 0.9510565162951535312, 1.000000000000000000, 0.9510565162951535312, 1.000000000000000000, 0.9510565162951535312, 1.000000000000000000, 0.9510565162951535312, 1.000000000000000000, 0.9510565162951535312, 1.000000000000000000, 0.9510565162951535312, 1.000000000000000000, 0.9510565162951535312, 1.000000000000000000, 0.9510565162951535312, 1.000000000000000000, 0.9510565162951535312, 1.000000000000000000, 0.9510565162951535312, 1.000000000000000000, 0.9510565162951535312, 1.000000000000000000, 0.9510565162951535312, 1.000000000000000000),
 ( 1.000000000000000000, 0.9510565162951535312, 1.000000000000000000, 0.9510565162951535312, 1.000000000000000000, 0.9510565162951535312, 1.000000000000000000, 0.9510565162951535312, 1.000000000000000000, 0.9510565162951535312, 1.000000000000000000, 0.9510565162951535312, 1.000000000000000000, 0.9510565162951535312, 1.000000000000000000, 0.9510565162951535312, 1.000000000000000000, 0.9510565162951535312, 1.000000000000000000, 0.9510565162951535312, 1.000000000000000000, 0.9510565162951535312, 1.000000000000000000, 0.9510565162951535312, 1.000000000000000000, 0.9510565162951535312, 1.000000000000000000, 0.9510565162951535312, 1.000000000000000000, 0.9510565162951535312, 1.000000000000000000, 0.9510565162951535312, 1.000000000000000000, 0.9510565162951535312, 1.000000000000000000, 0.9510565162951535312, 1.000000000000000000, 0.9510565162951535312, 1.000000000000000000, 0.9510565162951535312, 1.000000000000000000, 0.9510565162951535312, 1.000000000000000000, 0.9510565162951535312, 1.000000000000000000, 0.9510565162951535312, 1.000000000000000000, 0.9510565162951535312, 1.000000000000000000, 0.9510565162951535312, 1.000000000000000000, 0.9510565162951535312, 1.000000000000000000, 0.9510565162951535312, 1.000000000000000000, 0.9510565162951535312, 1.000000000000000000, 0.9510565162951535312, 1.000000000000000000, 0.9510565162951535312, 1.000000000000000000, 0.9510565162951535312, 1.000000000000000000, 0.9510565162951535312, 1.000000000000000000, 0.9510565162951535312, 1.000000000000000000, 0.9510565162951535312, 1.000000000000000000, 0.9510565162951535312, 1.000000000000000000, 0.9510565162951535312, 1.000000000000000000, 0.9510565162951535312, 1.000000000000000000, 0.9510565162951535312, 1.000000000000000000, 0.9510565162951535312, 1.000000000000000000, 0.9510565162951535312, 1.000000000000000000, 0.9510565162951535312, 1.000000000000000000, 0.9510565162951535312, 1.000000000000000000, 0.9510565162951535312, 1.000000000000000000, 0.9510565162951535312, 1.000000000000000000, 0.9510565162951535312, 1.000000000000000000, 0.9510565162951535312, 1.000000000000000000, 0.9510565162951535312, 1.000000000000000000, 0.9510565162951535312, 1.000000000000000000, 0.9510565162951535312, 1.000000000000000000, 0.9510565162951535312, 1.000000000000000000, 0.9510565162951535312, 1.000000000000000000, 0.9510565162951535312, 1.000000000000000000, 0.9510565162951535312, 1.000000000000000000, 0.9510565162951535312, 1.000000000000000000, 0.9510565162951535312, 1.000000000000000000, 0.9510565162951535312, 1.000000000000000000, 0.9510565162951535312, 1.000000000000000000, 0.9510565162951535312, 1.000000000000000000, 0.9510565162951535312, 1.000000000000000000, 0.9510565162951535312, 1.000000000000000000, 0.9510565162951535312, 1.000000000000000000, 0.9510565162951535312, 1.000000000000000000, 0.9510565162951535312, 1.000000000000000000, 0.9510565162951535312, 1.000000000000000000, 0.9510565162951535312, 1.000000000000000000, 0.9510565162951535312, 1.000000000000000000, 0.9510565162951535312, 1.000000000000000000, 0.9510565162951535312, 1.000000000000000000, 0.9510565162951535312, 1.000000000000000000, 0.9510565162951535312, 1.000000000000000000, 0.9510565162951535312, 1.000000000000000000, 0.9510565162951535312, 1.000000000000000000, 0.9510565162951535312, 1.000000000000000000, 0.9510565162951535312, 1.000000000000000000, 0.9510565162951535312, 1.000000000000000000, 0.9510565162951535312, 1.000000000000000000, 0.9510565162951535312, 1.000000000000000000, 0.9510565162951535312, 1.000000000000000000, 0.9510565162951535312, 1.000000000000000000, 0.9510565162951535312, 1.000000000000000000, 0.9510565162951535312, 1.000000000000000000, 0.9510565162951535312, 1.000000000000000000, 0.9510565162951535312, 1.000000000000000000, 0.9510565162951535312, 1.000000000000000000, 0.9510565162951535312, 1.000000000000000000, 0.9510565162951535312, 1.000000000000000000, 0.9510565162951535312, 1.000000000000000000, 0.9510565162951535312, 1.000000000000000000, 0.9510565162951535312, 1.000000000000000000, 0.9510565162951535312, 1.000000000000000000) ) ) 
 REPRESENTATION_ITEM ( '' )  SURFACE ( )  );
#2681=ADVANCED_FACE ( 'NONE', ( #33276, #14755 ), #20772, .F. ) ;
#2685=CARTESIAN_POINT ( 'NONE',  ( -23.41746825000000598, 6.224999997268799490, 7.608796670333726198 ) ) ;
#2706=DIRECTION ( 'NONE',  ( 0.000000000000000000, -1.000000000000000000, 0.000000000000000000 ) ) ;
#2716=CYLINDRICAL_SURFACE ( 'NONE', #25592, 24.50000000000000000 ) ;
#2727=ORIENTED_EDGE ( 'NONE', *, *, #33353, .T. ) ;
#2732=ORIENTED_EDGE ( 'NONE', *, *, #3020, .F. ) ;
#2743=CARTESIAN_POINT ( 'NONE',  ( -24.50000000000000000, 7.000000000000006217, -3.000384657911015469E-15 ) ) ;
#2751=CARTESIAN_POINT ( 'NONE',  ( 24.50000000000000000, 9.749999994537628112, 0.000000000000000000 ) ) ;
#2769=CARTESIAN_POINT ( 'NONE',  ( -23.41746824999999887, 12.12499999726882116, -2.867812753649727150E-15 ) ) ;
#2785=CARTESIAN_POINT ( 'NONE',  ( 18.94512977948575738, 2.424999997268806329, 13.76444248337723408 ) ) ;
#2794=CARTESIAN_POINT ( 'NONE',  ( -7.236395654485757944, 17.72499999726881370, -22.27133577429736988 ) ) ;
#2806=CARTESIAN_POINT ( 'NONE',  ( -23.41746824999999887, 11.62499999726881938, -2.867812753649727150E-15 ) ) ;
#2810=LINE ( 'NONE', #26980, #2022 ) ;
#2827=CARTESIAN_POINT ( 'NONE',  ( -24.50000000000000000, 14.89999999999999503, -7.960532557706207157 ) ) ;
#2832=CARTESIAN_POINT ( 'NONE',  ( -24.50000000000000355, 18.64999999453763380, -7.960532557706207157 ) ) ;
#2840=CARTESIAN_POINT ( 'NONE',  ( -3.880418787951136483, 6.551254281546842861, -24.50000000000000000 ) ) ;
#2847=CARTESIAN_POINT ( 'NONE',  ( -23.41746825000000598, 10.22499999726881903, 7.608796670333726198 ) ) ;
#2863=EDGE_CURVE ( 'NONE', #24126, #29527, #11362, .T. ) ;
#2876=CARTESIAN_POINT ( 'NONE',  ( -1.756012107511856980E-14, 6.249999994537623671, -24.50000000000000000 ) ) ;
#2891=CARTESIAN_POINT ( 'NONE',  ( -3.880418787951174675, 12.30125427608447275, -24.49999999999998579 ) ) ;
#2900=ORIENTED_EDGE ( 'NONE', *, *, #181, .F. ) ;
#2917=CARTESIAN_POINT ( 'NONE',  ( -15.14183272437241889, 8.700000000000017053, -20.84094480462497856 ) ) ;
#2924=CARTESIAN_POINT ( 'NONE',  ( 24.50000000000000000, 9.649999994537628467, 7.960532557706212486 ) ) ;
#2939=CARTESIAN_POINT ( 'NONE',  ( 23.41746824999999887, 11.22499999726881548, -7.608796670333727974 ) ) ;
#2956=CARTESIAN_POINT ( 'NONE',  ( -18.94512977948575738, 7.424999997268811214, -13.76444248337723231 ) ) ;
#2967=CARTESIAN_POINT ( 'NONE',  ( -23.41746825000000243, 18.02499999726880731, -7.608796670333730638 ) ) ;
#2981=CARTESIAN_POINT ( 'NONE',  ( 23.41746824999999887, 18.62499999726882649, 0.000000000000000000 ) ) ;
#2982=FACE_OUTER_BOUND ( 'NONE', #23459, .T. ) ;
#2983=ORIENTED_EDGE ( 'NONE', *, *, #609, .F. ) ;
#3007=CARTESIAN_POINT ( 'NONE',  ( -24.50000000000000000, 16.74999999453763522, -3.000384657911015469E-15 ) ) ;
#3020=EDGE_CURVE ( 'NONE', #33486, #14415, #23846, .T. ) ;
#3021=CARTESIAN_POINT ( 'NONE',  ( -18.94512977948575738, 13.92499999726881654, -13.76444248337723231 ) ) ;
#3022=VECTOR ( 'NONE', #33435, 1000.000000000000000 ) ;
#3039=AXIS2_PLACEMENT_3D ( 'NONE', #4768, #14730, #15246 ) ;
#3058=CARTESIAN_POINT ( 'NONE',  ( -4.223320258572819786E-15, 11.24999999453762456, 24.50000000000000000 ) ) ;
#3064=CIRCLE ( 'NONE', #11810, 15.00000000000000000 ) ;
#3067=CARTESIAN_POINT ( 'NONE',  ( -19.82091636218621034, 12.80000000000000604, -14.40073868116559552 ) ) ;
#3088=CARTESIAN_POINT ( 'NONE',  ( -15.14183272437241889, 2.700000000000001954, -20.84094480462497856 ) ) ;
#3094=CARTESIAN_POINT ( 'NONE',  ( 23.41746824999999887, 2.724999997268822138, -7.608796670333727974 ) ) ;
#3108=DIRECTION ( 'NONE',  ( -0.000000000000000000, -1.000000000000000000, -0.000000000000000000 ) ) ;
#3112=CARTESIAN_POINT ( 'NONE',  ( 18.94512977948576093, 15.32499999726880091, -13.76444248337722875 ) ) ;
#3127=CARTESIAN_POINT ( 'NONE',  ( 1.507698388325705758E-15, 3.124999997268809615, -24.62258325217400312 ) ) ;
#3135=AXIS2_PLACEMENT_3D ( 'NONE', #6451, #6110, #16590 ) ;
#3149=CARTESIAN_POINT ( 'NONE',  ( -7.236395654485763274, 14.02499999726880553, 22.27133577429736633 ) ) ;
#3167=CARTESIAN_POINT ( 'NONE',  ( -1.756012107511856980E-14, 2.500000000000005773, -24.50000000000000000 ) ) ;
#3177=CARTESIAN_POINT ( 'NONE',  ( -24.50000000000001066, 16.84999999453763309, 7.960532557706201828 ) ) ;
#3188=CARTESIAN_POINT ( 'NONE',  ( 3.445340210940985210E-14, 7.249999994537621895, 24.50000000000000000 ) ) ;
#3190=CARTESIAN_POINT ( 'NONE',  ( -18.94512977948575738, 17.92499999726882010, -13.76444248337723231 ) ) ;
#3232=CARTESIAN_POINT ( 'NONE',  ( -24.50000000000000000, 12.90000000000000036, -7.960532557706207157 ) ) ;
#3235=ORIENTED_EDGE ( 'NONE', *, *, #181, .T. ) ;
#3251=CARTESIAN_POINT ( 'NONE',  ( -19.82091636218621389, 11.19999999999998863, 14.40073868116558842 ) ) ;
#3253=CARTESIAN_POINT ( 'NONE',  ( -7.570916362186210335, 4.349999994537640191, -23.30088464923126779 ) ) ;
#3255=CARTESIAN_POINT ( 'NONE',  ( 1.507698388325705758E-15, 1.124999997268814722, -24.62258325217400312 ) ) ;
#3259=CARTESIAN_POINT ( 'NONE',  ( 23.11635443782376242, 16.99999999999997868, -3.820720850812610259 ) ) ;
#3273=CARTESIAN_POINT ( 'NONE',  ( 20.58269335310955839, 16.96161537386475260, 11.51052958701926698 ) ) ;
#3287=EDGE_CURVE ( 'NONE', #11786, #24787, #21809, .T. ) ;
#3291=CARTESIAN_POINT ( 'NONE',  ( 18.94512977948576093, 4.824999997268819563, -13.76444248337722875 ) ) ;
#3300=CARTESIAN_POINT ( 'NONE',  ( 14.47279130897151589, 18.82499999726881157, 19.92008829642072953 ) ) ;
#3302=CARTESIAN_POINT ( 'NONE',  ( -7.579748464070167083E-14, 10.49999999999999112, -24.50000000000000000 ) ) ;
#3314=CARTESIAN_POINT ( 'NONE',  ( -14.47279130897152122, 17.92499999726880588, 19.92008829642072243 ) ) ;
#3318=CARTESIAN_POINT ( 'NONE',  ( 1.555960095263670572E-15, 12.50000000000000355, -24.50000000000000000 ) ) ;
#3336=ORIENTED_EDGE ( 'NONE', *, *, #20704, .F. ) ;
#3337=CARTESIAN_POINT ( 'NONE',  ( 14.47279130897151589, 2.824999997268819119, 19.92008829642072953 ) ) ;
#3342=PRODUCT_DEFINITION_SHAPE ( 'NONE', 'NONE',  #16263 ) ;
#3349=CARTESIAN_POINT ( 'NONE',  ( 0.000000000000000000, -22.99999999999999289, 0.000000000000000000 ) ) ;
#3352=CARTESIAN_POINT ( 'NONE',  ( 0.000000000000000000, -22.99999999999999289, 0.000000000000000000 ) ) ;
#3354=CARTESIAN_POINT ( 'NONE',  ( -23.41746824999999887, 14.12499999726882294, -2.867812753649727150E-15 ) ) ;
#3378=CARTESIAN_POINT ( 'NONE',  ( -19.82091636218621389, 16.94999999453764161, 14.40073868116558842 ) ) ;
#3386=CARTESIAN_POINT ( 'NONE',  ( 15.62859546567362656, 16.99999999999999645, 17.78191404720239888 ) ) ;
#3415=CARTESIAN_POINT ( 'NONE',  ( 7.570916362186207671, 9.599999999999997868, 23.30088464923126779 ) ) ;
#3418=CARTESIAN_POINT ( 'NONE',  ( 18.94512977948575738, 10.42499999726881299, 13.76444248337723408 ) ) ;
#3419=CARTESIAN_POINT ( 'NONE',  ( 24.50000000000000000, 4.099999999999986322, -7.960532557706203605 ) ) ;
#3433=CARTESIAN_POINT ( 'NONE',  ( -3.880418787951174675, 16.55125428154684997, -24.49999999999998579 ) ) ;
#3453=CARTESIAN_POINT ( 'NONE',  ( -18.94512977948575738, 9.424999997268812990, -13.76444248337723231 ) ) ;
#3475=CARTESIAN_POINT ( 'NONE',  ( 18.94512977948575738, 16.42499999726882010, 13.76444248337723408 ) ) ;
#3479=DIRECTION ( 'NONE',  ( 0.000000000000000000, -1.000000000000000000, 0.000000000000000000 ) ) ;
#3482=ORIENTED_EDGE ( 'NONE', *, *, #21089, .T. ) ;
#3485=ADVANCED_FACE ( 'NONE', ( #18956 ), #29724, .T. ) ;
#3488=CARTESIAN_POINT ( 'NONE',  ( -19.82091636218621389, 2.949999994537627401, 14.40073868116558842 ) ) ;
#3495=( NAMED_UNIT ( * ) PLANE_ANGLE_UNIT ( ) SI_UNIT ( $, .RADIAN. ) );
#3501=CARTESIAN_POINT ( 'NONE',  ( -14.47279130897151589, 3.824999997268816454, -19.92008829642072598 ) ) ;
#3517=CARTESIAN_POINT ( 'NONE',  ( 18.94512977948575738, 16.92499999726882010, 13.76444248337723408 ) ) ;
#3518=VERTEX_POINT ( 'NONE', #1229 ) ;
#3547=CARTESIAN_POINT ( 'NONE',  ( 17.67679332509665713, 16.99999999999998224, 15.66627074469097458 ) ) ;
#3557=CARTESIAN_POINT ( 'NONE',  ( -7.570916362186215665, 13.39999999999999503, 23.30088464923126423 ) ) ;
#3564=ADVANCED_FACE ( 'NONE', ( #26994 ), #8798, .F. ) ;
#3582=CARTESIAN_POINT ( 'NONE',  ( -19.82091636218621389, 9.200000000000013500, 14.40073868116558842 ) ) ;
#3586=CARTESIAN_POINT ( 'NONE',  ( 23.41746824999999887, 8.624999997268817609, 0.000000000000000000 ) ) ;
#3590=CARTESIAN_POINT ( 'NONE',  ( 15.14183272437242422, 2.049999994537635484, -20.84094480462497856 ) ) ;
#3621=CARTESIAN_POINT ( 'NONE',  ( 14.47279130897151767, 8.924999997268800556, -19.92008829642072598 ) ) ;
#3641=CARTESIAN_POINT ( 'NONE',  ( -18.94512977948575738, 17.42499999726882010, -13.76444248337723231 ) ) ;
#3656=VECTOR ( 'NONE', #10313, 1000.000000000000000 ) ;
#3668=CARTESIAN_POINT ( 'NONE',  ( 18.94512977948576093, 9.324999997268824004, -13.76444248337722875 ) ) ;
#3683=CARTESIAN_POINT ( 'NONE',  ( 7.236395654485755280, 12.72499999726881015, 22.27133577429736988 ) ) ;
#3709=CARTESIAN_POINT ( 'NONE',  ( -18.67342709957029001, 16.97452379773154973, 15.98012215616494913 ) ) ;
#3718=CARTESIAN_POINT ( 'NONE',  ( 7.570916362186207671, 11.34999999453761887, 23.30088464923126779 ) ) ;
#3725=FACE_OUTER_BOUND ( 'NONE', #17369, .T. ) ;
#3731=VERTEX_POINT ( 'NONE', #3167 ) ;
#3749=CARTESIAN_POINT ( 'NONE',  ( 19.82091636218621034, 13.80000000000000604, 14.40073868116559730 ) ) ;
#3753=CARTESIAN_POINT ( 'NONE',  ( 23.41746824999999887, 10.72499999726880127, -7.608796670333727974 ) ) ;
#3754=CARTESIAN_POINT ( 'NONE',  ( 24.50000000000000000, 3.749999994537622783, 0.000000000000000000 ) ) ;
#3759=CARTESIAN_POINT ( 'NONE',  ( 3.445340210940985210E-14, 9.249999994537636994, 24.50000000000000000 ) ) ;
#3783=CARTESIAN_POINT ( 'NONE',  ( 15.14183272437242067, 11.70000000000000817, 20.84094480462498211 ) ) ;
#3788=CARTESIAN_POINT ( 'NONE',  ( -23.41746825000000243, 9.524999997268810858, -7.608796670333730638 ) ) ;
#3813=CARTESIAN_POINT ( 'NONE',  ( -4.523095164977117273E-15, 4.624999997268820273, 24.62258325217400312 ) ) ;
#3826=DIRECTION ( 'NONE',  ( 0.000000000000000000, 0.000000000000000000, -1.000000000000000000 ) ) ;
#3833=CARTESIAN_POINT ( 'NONE',  ( 18.94512977948575738, 4.924999997268808549, 13.76444248337723408 ) ) ;
#3842=CARTESIAN_POINT ( 'NONE',  ( 24.50000000000000000, 5.899999999999987921, 7.960532557706212486 ) ) ;
#3845=CARTESIAN_POINT ( 'NONE',  ( 1.555960095263670572E-15, 8.249999994537619230, -24.50000000000000000 ) ) ;
#3847=CARTESIAN_POINT ( 'NONE',  ( -4.523095164977116484E-15, 2.124999997268812280, 24.62258325217400312 ) ) ;
#3853=( BOUNDED_CURVE ( )  B_SPLINE_CURVE ( 2, ( #30289, #17442, #6791, #29957, #16935, #33204, #9355, #17268, #15038, #20188, #27731, #27393, #4559 ),
 .UNSPECIFIED., .F., .T. ) 
 B_SPLINE_CURVE_WITH_KNOTS ( ( 3, 2, 2, 2, 2, 2, 3 ),
 ( 0.08333333333333334259, 0.08888888888888889228, 0.1000000000000000056, 0.1111111111111111049, 0.1222222222222222321, 0.1333333333333333315, 0.1388888888888888951 ),
 .UNSPECIFIED. ) 
 CURVE ( )  GEOMETRIC_REPRESENTATION_ITEM ( )  RATIONAL_B_SPLINE_CURVE ( ( 0.9755282581475768211, 0.9755282581475768211, 1.000000000000000000, 0.9510565162951535312, 1.000000000000000000, 0.9510565162951535312, 1.000000000000000000, 0.9510565162951535312, 1.000000000000000000, 0.9510565162951535312, 1.000000000000000000, 0.9755282581475767101, 0.9755282581475768211 ) ) 
 REPRESENTATION_ITEM ( '' )  );
#3858=ORIENTED_EDGE ( 'NONE', *, *, #31876, .F. ) ;
#3873=CARTESIAN_POINT ( 'NONE',  ( 24.50000000000000000, 7.749999994537626336, 0.000000000000000000 ) ) ;
#3880=CARTESIAN_POINT ( 'NONE',  ( -16.57479016809132588, 16.99999999999998579, 18.03908112418252685 ) ) ;
#3883=LINE ( 'NONE', #17103, #23419 ) ;
#3888=CARTESIAN_POINT ( 'NONE',  ( -7.570916362186210335, 10.34999999453761710, -23.30088464923126779 ) ) ;
#3898=ORIENTED_EDGE ( 'NONE', *, *, #10326, .T. ) ;
#3901=CARTESIAN_POINT ( 'NONE',  ( 1.555960095263670572E-15, 16.24999999453762101, -24.50000000000000000 ) ) ;
#3916=CARTESIAN_POINT ( 'NONE',  ( 15.14183272437242245, 10.29999999999999361, -20.84094480462497856 ) ) ;
#3920=CARTESIAN_POINT ( 'NONE',  ( 1.507698388325705758E-15, 13.12499999726881228, -24.62258325217400312 ) ) ;
#3924=CARTESIAN_POINT ( 'NONE',  ( -9.163862182818718338, 16.99999999999998224, -22.02512863723370629 ) ) ;
#3953=CARTESIAN_POINT ( 'NONE',  ( 23.41746825000000243, 10.52499999726880731, 7.608796670333735079 ) ) ;
#3979=CARTESIAN_POINT ( 'NONE',  ( 18.94512977948575738, 2.924999997268806773, 13.76444248337723408 ) ) ;
#3997=CARTESIAN_POINT ( 'NONE',  ( 7.570916362186207671, 7.599999999999996092, 23.30088464923126779 ) ) ;
#4000=ORIENTED_EDGE ( 'NONE', *, *, #12601, .T. ) ;
#4001=CARTESIAN_POINT ( 'NONE',  ( -4.523095164977116484E-15, 6.624999997268815832, 24.62258325217400312 ) ) ;
#4012=CARTESIAN_POINT ( 'NONE',  ( 15.14183272437242067, 7.449999994537640724, 20.84094480462498211 ) ) ;
#4014=AXIS2_PLACEMENT_3D ( 'NONE', #3352, #26856, #13822 ) ;
#4015=CARTESIAN_POINT ( 'NONE',  ( 18.94512977948575738, 18.92499999726882010, 13.76444248337723408 ) ) ;
#4039=CARTESIAN_POINT ( 'NONE',  ( -24.50000000000000355, 6.649999994537636461, -7.960532557706207157 ) ) ;
#4052=( BOUNDED_CURVE ( )  B_SPLINE_CURVE ( 2, ( #15406, #31347, #30656, #25862, #2529, #7326, #33231, #26035, #28097, #12997, #4585, #17810, #33765 ),
 .UNSPECIFIED., .F., .F. ) 
 B_SPLINE_CURVE_WITH_KNOTS ( ( 3, 2, 2, 2, 2, 2, 3 ),
 ( 0.2500000000000000000, 0.2555555555555555358, 0.2666666666666666630, 0.2777777777777777901, 0.2888888888888888618, 0.2999999999999999889, 0.3055555555555555802 ),
 .UNSPECIFIED. ) 
 CURVE ( )  GEOMETRIC_REPRESENTATION_ITEM ( )  RATIONAL_B_SPLINE_CURVE ( ( 0.9755282581475768211, 0.9755282581475768211, 1.000000000000000000, 0.9510565162951535312, 1.000000000000000000, 0.9510565162951535312, 1.000000000000000000, 0.9510565162951535312, 1.000000000000000000, 0.9510565162951535312, 1.000000000000000000, 0.9755282581475765991, 0.9755282581475767101 ) ) 
 REPRESENTATION_ITEM ( '' )  );
#4053=CARTESIAN_POINT ( 'NONE',  ( -7.236395654485763274, 4.524999997268825069, 22.27133577429736633 ) ) ;
#4055=DIRECTION ( 'NONE',  ( 0.000000000000000000, -1.000000000000000000, 0.000000000000000000 ) ) ;
#4083=CARTESIAN_POINT ( 'NONE',  ( 24.50000000000000355, 17.89999999999998437, 7.960532557706212486 ) ) ;
#4087=CARTESIAN_POINT ( 'NONE',  ( -23.41746824999999887, 13.52499999726880198, -7.608796670333730638 ) ) ;
#4091=CARTESIAN_POINT ( 'NONE',  ( -1.756012107511856980E-14, 4.249999994537631665, -24.50000000000000000 ) ) ;
#4106=CIRCLE ( 'NONE', #23308, 24.50000000000000000 ) ;
#4123=CARTESIAN_POINT ( 'NONE',  ( 24.50000000000000000, 0.000000000000000000, 0.000000000000000000 ) ) ;
#4148=CARTESIAN_POINT ( 'NONE',  ( 7.236395654485760609, 1.524999997268822183, -22.27133577429736633 ) ) ;
#4151=ORIENTED_EDGE ( 'NONE', *, *, #17536, .T. ) ;
#4173=CARTESIAN_POINT ( 'NONE',  ( 18.94512977948576093, 5.324999997268820451, -13.76444248337722875 ) ) ;
#4187=CARTESIAN_POINT ( 'NONE',  ( 18.94512977948575738, 2.424999997268806329, 13.76444248337723408 ) ) ;
#4211=CARTESIAN_POINT ( 'NONE',  ( 19.82091636218621034, 5.549999994537619052, 14.40073868116559730 ) ) ;
#4226=CARTESIAN_POINT ( 'NONE',  ( -4.223320258572819786E-15, 11.24999999453762456, 24.50000000000000000 ) ) ;
#4251=CARTESIAN_POINT ( 'NONE',  ( -19.82091636218621389, 17.19999999999999218, 14.40073868116558842 ) ) ;
#4256=CARTESIAN_POINT ( 'NONE',  ( 1.507698388325705758E-15, 15.12499999726880873, -24.62258325217400312 ) ) ;
#4260=CARTESIAN_POINT ( 'NONE',  ( 23.12028783339972549, 16.99999999999998934, 3.796702233379605662 ) ) ;
#4290=CARTESIAN_POINT ( 'NONE',  ( 19.82091636218621389, 2.200000000000007283, -14.40073868116559197 ) ) ;
#4318=ORIENTED_EDGE ( 'NONE', *, *, #15607, .T. ) ;
#4319=EDGE_CURVE ( 'NONE', #13996, #23373, #26358, .T. ) ;
#4322=ORIENTED_EDGE ( 'NONE', *, *, #20163, .T. ) ;
#4340=CARTESIAN_POINT ( 'NONE',  ( 1.507698388325705758E-15, 5.624999997268818497, -24.62258325217400312 ) ) ;
#4353=CARTESIAN_POINT ( 'NONE',  ( -14.47279130897151589, 1.324999997268808238, -19.92008829642072598 ) ) ;
#4362=ORIENTED_EDGE ( 'NONE', *, *, #28129, .F. ) ;
#4365=ORIENTED_EDGE ( 'NONE', *, *, #17881, .F. ) ;
#4378=CARTESIAN_POINT ( 'NONE',  ( 15.14183272437241889, 3.449999994537620296, 20.84094480462498211 ) ) ;
#4393=CARTESIAN_POINT ( 'NONE',  ( 23.41746825000000243, 3.224999997268806151, -7.608796670333727974 ) ) ;
#4405=CARTESIAN_POINT ( 'NONE',  ( -3.880418787951124493, 9.198745712990794132, 24.50000000000000355 ) ) ;
#4421=CARTESIAN_POINT ( 'NONE',  ( -7.570916362186215665, 17.39999999999999858, 23.30088464923126423 ) ) ;
#4426=CARTESIAN_POINT ( 'NONE',  ( 18.94512977948576093, 16.82499999726880091, -13.76444248337722875 ) ) ;
#4461=CARTESIAN_POINT ( 'NONE',  ( 18.94512977948575738, 18.42499999726882010, 13.76444248337723408 ) ) ;
#4478=CARTESIAN_POINT ( 'NONE',  ( 7.570916362186207671, 15.60000000000000320, 23.30088464923126779 ) ) ;
#4487=CARTESIAN_POINT ( 'NONE',  ( 18.94512977948576093, 5.324999997268820451, -13.76444248337722875 ) ) ;
#4501=CARTESIAN_POINT ( 'NONE',  ( 23.41746825000000243, 0.7249999972688272454, -7.608796670333727974 ) ) ;
#4511=CARTESIAN_POINT ( 'NONE',  ( 18.94512977948575738, 10.92499999726881299, 13.76444248337723408 ) ) ;
#4518=DIRECTION ( 'NONE',  ( 0.000000000000000000, -1.000000000000000000, 0.000000000000000000 ) ) ;
#4525=CARTESIAN_POINT ( 'NONE',  ( -14.47279130897152122, 18.42499999726882365, 19.92008829642072243 ) ) ;
#4550=CARTESIAN_POINT ( 'NONE',  ( -7.570916362186210335, 12.34999999453761887, -23.30088464923126779 ) ) ;
#4559=CARTESIAN_POINT ( 'NONE',  ( -1.756012107511856980E-14, 2.500000000000005773, -24.50000000000000000 ) ) ;
#4577=CARTESIAN_POINT ( 'NONE',  ( -4.223320258572819786E-15, 9.499999999999992895, 24.50000000000000000 ) ) ;
#4585=CARTESIAN_POINT ( 'NONE',  ( -7.570916362186215665, 5.399999999999987921, 23.30088464923126423 ) ) ;
#4593=CARTESIAN_POINT ( 'NONE',  ( -24.50000000000001066, 17.09999999999998366, 7.960532557706201828 ) ) ;
#4601=CARTESIAN_POINT ( 'NONE',  ( -24.48923876278562517, 16.99999999999998579, -0.4945881427486832349 ) ) ;
#4630=SURFACE_STYLE_USAGE ( .BOTH. , #14762 ) ;
#4633=CARTESIAN_POINT ( 'NONE',  ( 14.47279130897151589, 18.32499999726882578, 19.92008829642072953 ) ) ;
#4639=ORIENTED_EDGE ( 'NONE', *, *, #30160, .F. ) ;
#4659=CARTESIAN_POINT ( 'NONE',  ( 23.41746824999999887, 11.12499999726881938, 0.000000000000000000 ) ) ;
#4666=CARTESIAN_POINT ( 'NONE',  ( 24.50000000000000000, 5.749999994537624559, 0.000000000000000000 ) ) ;
#4683=CARTESIAN_POINT ( 'NONE',  ( -23.41746825000000243, 16.02499999726881086, -7.608796670333730638 ) ) ;
#4684=CARTESIAN_POINT ( 'NONE',  ( -18.94512977948575738, 1.424999997268805441, -13.76444248337723231 ) ) ;
#4696=CARTESIAN_POINT ( 'NONE',  ( 18.94512977948576093, 6.824999997268821339, -13.76444248337722875 ) ) ;
#4697=CARTESIAN_POINT ( 'NONE',  ( -4.223320258572819786E-15, 13.50000000000000355, 24.50000000000000000 ) ) ;
#4706=EDGE_LOOP ( 'NONE', ( #2983, #19651, #11954, #25514 ) ) ;
#4720=CARTESIAN_POINT ( 'NONE',  ( 15.14183272437242245, 16.04999999453762882, -20.84094480462497856 ) ) ;
#4768=CARTESIAN_POINT ( 'NONE',  ( 0.000000000000000000, 16.99999999999998579, 0.000000000000000000 ) ) ;
#4777=DIRECTION ( 'NONE',  ( 0.000000000000000000, 0.000000000000000000, -1.000000000000000000 ) ) ;
#4798=CARTESIAN_POINT ( 'NONE',  ( 3.880418787951140036, 14.19874571299077637, -24.49999999999999645 ) ) ;
#4802=CARTESIAN_POINT ( 'NONE',  ( -24.50000000000000355, 0.9000000000000005773, -7.960532557706207157 ) ) ;
#4818=CARTESIAN_POINT ( 'NONE',  ( 19.82091636218621034, 15.80000000000000782, 14.40073868116559730 ) ) ;
#4828=CARTESIAN_POINT ( 'NONE',  ( 23.41746824999999887, 5.124999997268814056, 0.000000000000000000 ) ) ;
#4837=DIRECTION ( 'NONE',  ( 0.000000000000000000, -1.000000000000000000, 0.000000000000000000 ) ) ;
#4856=CARTESIAN_POINT ( 'NONE',  ( -14.47279130897151589, 11.82499999726882578, -19.92008829642072598 ) ) ;
#4857=CARTESIAN_POINT ( 'NONE',  ( -4.523095164977117273E-15, 4.124999997268806951, 24.62258325217400312 ) ) ;
#4870=CARTESIAN_POINT ( 'NONE',  ( 14.47279130897151589, 6.324999997268824892, 19.92008829642072953 ) ) ;
#4871=CARTESIAN_POINT ( 'NONE',  ( 15.14183272437242067, 13.70000000000000462, 20.84094480462498211 ) ) ;
#4880=ORIENTED_EDGE ( 'NONE', *, *, #12497, .T. ) ;
#4893=EDGE_CURVE ( 'NONE', #29527, #17796, #10273, .T. ) ;
#4894=CARTESIAN_POINT ( 'NONE',  ( 15.14183272437242245, 10.04999999453761639, -20.84094480462497856 ) ) ;
#4907=CARTESIAN_POINT ( 'NONE',  ( -7.236395654485763274, 6.524999997268826846, 22.27133577429736633 ) ) ;
#4913=VERTEX_POINT ( 'NONE', #32202 ) ;
#4918=CARTESIAN_POINT ( 'NONE',  ( 3.880418787951134707, 9.551254281546839309, 24.50000000000000000 ) ) ;
#4920=CARTESIAN_POINT ( 'NONE',  ( -24.50000000000000000, 8.649999994537632020, -7.960532557706207157 ) ) ;
#4939=CARTESIAN_POINT ( 'NONE',  ( 14.47279130897151944, 14.92499999726881477, -19.92008829642072598 ) ) ;
#4946=CARTESIAN_POINT ( 'NONE',  ( -7.579748464070165821E-14, 12.24999999453762456, -24.50000000000000000 ) ) ;
#4978=CARTESIAN_POINT ( 'NONE',  ( 15.14183272437241889, 7.699999999999988631, 20.84094480462498211 ) ) ;
#4986=CARTESIAN_POINT ( 'NONE',  ( 24.50000000000000000, 9.849999994537622428, -7.960532557706203605 ) ) ;
#4995=CARTESIAN_POINT ( 'NONE',  ( -6.668400408272875007E-16, 0.5000000000000068834, -24.50000000000000355 ) ) ;
#4999=CARTESIAN_POINT ( 'NONE',  ( -23.41746825000000243, 6.224999997268798602, 7.608796670333725309 ) ) ;
#5025=CARTESIAN_POINT ( 'NONE',  ( 23.41746824999999887, 15.12499999726882294, 0.000000000000000000 ) ) ;
#5026=CARTESIAN_POINT ( 'NONE',  ( 23.41746824999999887, 2.524999997268799312, 7.608796670333735079 ) ) ;
#5032=UNCERTAINTY_MEASURE_WITH_UNIT (LENGTH_MEASURE( 1.000000000000000082E-05 ), #17682, 'distance_accuracy_value', 'NONE');
#5039=CARTESIAN_POINT ( 'NONE',  ( 18.94512977948575738, 12.42499999726881477, 13.76444248337723408 ) ) ;
#5064=CARTESIAN_POINT ( 'NONE',  ( 24.50000000000000355, 13.84999999453761177, -7.960532557706203605 ) ) ;
#5072=CARTESIAN_POINT ( 'NONE',  ( -24.50000000000000711, 7.100000000000008527, 7.960532557706201828 ) ) ;
#5080=CARTESIAN_POINT ( 'NONE',  ( 7.236395654485755280, 10.72499999726880837, 22.27133577429736988 ) ) ;
#5116=DIRECTION ( 'NONE',  ( 0.000000000000000000, 0.000000000000000000, -1.000000000000000000 ) ) ;
#5146=CARTESIAN_POINT ( 'NONE',  ( -24.50000000000001066, 7.100000000000007638, 7.960532557706201828 ) ) ;
#5165=FACE_OUTER_BOUND ( 'NONE', #24170, .T. ) ;
#5174=CARTESIAN_POINT ( 'NONE',  ( -18.94512977948575738, 7.924999997268811214, -13.76444248337723231 ) ) ;
#5192=CARTESIAN_POINT ( 'NONE',  ( 7.236395654485755280, 2.224999997268800378, 22.27133577429736988 ) ) ;
#5210=CARTESIAN_POINT ( 'NONE',  ( 24.50000000000000000, 0.000000000000000000, 0.000000000000000000 ) ) ;
#5212=CARTESIAN_POINT ( 'NONE',  ( 23.41746824999999887, 10.62499999726881938, 0.000000000000000000 ) ) ;
#5227=CARTESIAN_POINT ( 'NONE',  ( -3.880418787951146697, 6.301254276084462091, -24.49999999999999645 ) ) ;
#5237=CARTESIAN_POINT ( 'NONE',  ( 19.82091636218621389, 9.949999994537634507, -14.40073868116559197 ) ) ;
#5240=EDGE_CURVE ( 'NONE', #33508, #17247, #20307, .T. ) ;
#5246=CARTESIAN_POINT ( 'NONE',  ( 3.445340210940985210E-14, 7.499999999999994671, 24.50000000000000000 ) ) ;
#5253=CARTESIAN_POINT ( 'NONE',  ( -23.41746824999999887, 8.124999997268817609, -2.867812753649727150E-15 ) ) ;
#5256=VECTOR ( 'NONE', #30579, 1000.000000000000114 ) ;
#5280=EDGE_CURVE ( 'NONE', #6391, #17247, #29124, .T. ) ;
#5289=CARTESIAN_POINT ( 'NONE',  ( 7.168475036913831033, 16.99999999999999289, -22.36265383151947361 ) ) ;
#5316=ORIENTED_EDGE ( 'NONE', *, *, #15607, .F. ) ;
#5319=CARTESIAN_POINT ( 'NONE',  ( -15.14183272437241889, 4.699999999999995737, -20.84094480462497856 ) ) ;
#5337=CARTESIAN_POINT ( 'NONE',  ( 7.570916362186213000, 0.4000000000000114575, -23.30088464923126423 ) ) ;
#5343=CARTESIAN_POINT ( 'NONE',  ( 1.507698388325705758E-15, 11.62499999726880340, -24.62258325217400312 ) ) ;
#5353=DIRECTION ( 'NONE',  ( 0.000000000000000000, -0.000000000000000000, -1.000000000000000000 ) ) ;
#5359=CARTESIAN_POINT ( 'NONE',  ( -7.236395654485757944, 3.224999997268801266, -22.27133577429736988 ) ) ;
#5367=VERTEX_POINT ( 'NONE', #14694 ) ;
#5368=CARTESIAN_POINT ( 'NONE',  ( 1.507698388325705758E-15, 17.62499999726881938, -24.62258325217400312 ) ) ;
#5376=EDGE_CURVE ( 'NONE', #33486, #12563, #28952, .T. ) ;
#5382=CARTESIAN_POINT ( 'NONE',  ( -23.41746825000000243, 7.524999997268816188, -7.608796670333730638 ) ) ;
#5408=CARTESIAN_POINT ( 'NONE',  ( -7.570916362186215665, 19.14999999453761959, 23.30088464923126423 ) ) ;
#5422=CARTESIAN_POINT ( 'NONE',  ( -14.47279130897152122, 8.424999997268816543, 19.92008829642072243 ) ) ;
#5470=ADVANCED_FACE ( 'NONE', ( #33029 ), #30461, .T. ) ;
#5476=EDGE_CURVE ( 'NONE', #24093, #3731, #3853, .T. ) ;
#5488=CARTESIAN_POINT ( 'NONE',  ( 24.50000000000000355, 4.099999999999986322, -7.960532557706203605 ) ) ;
#5490=CARTESIAN_POINT ( 'NONE',  ( -15.14183272437242600, 3.049999994537633263, 20.84094480462497856 ) ) ;
#5496=CARTESIAN_POINT ( 'NONE',  ( 3.880418787951121828, 10.19874571299079413, -24.50000000000000355 ) ) ;
#5511=CARTESIAN_POINT ( 'NONE',  ( -18.94512977948576093, 16.32499999726880091, 13.76444248337722698 ) ) ;
#5512=EDGE_LOOP ( 'NONE', ( #21967, #5316, #10409, #9993 ) ) ;
#5529=CARTESIAN_POINT ( 'NONE',  ( -7.236395654485757944, 7.224999997268804819, -22.27133577429736988 ) ) ;
#5550=CARTESIAN_POINT ( 'NONE',  ( -18.94512977948576093, 17.82499999726880446, 13.76444248337722698 ) ) ;
#5556=AXIS2_PLACEMENT_3D ( 'NONE', #9940, #2206, #12685 ) ;
#5577=CARTESIAN_POINT ( 'NONE',  ( -15.14183272437242600, 19.04999999453762172, 20.84094480462497856 ) ) ;
#5591=CARTESIAN_POINT ( 'NONE',  ( 23.41746825000000243, 15.02499999726881086, 7.608796670333735079 ) ) ;
#5627=DIRECTION ( 'NONE',  ( 0.000000000000000000, -1.000000000000000000, 0.000000000000000000 ) ) ;
#5656=CARTESIAN_POINT ( 'NONE',  ( 15.14183272437242245, 6.300000000000004263, -20.84094480462497856 ) ) ;
#5661=CARTESIAN_POINT ( 'NONE',  ( -23.41746824999999887, 3.624999997268813168, -2.867812753649727150E-15 ) ) ;
#5662=CARTESIAN_POINT ( 'NONE',  ( 3.880418787951132042, 4.448745718453150033, -24.50000000000000355 ) ) ;
#5671=ADVANCED_FACE ( 'NONE', ( #594 ), #13664, .T. ) ;
#5683=CARTESIAN_POINT ( 'NONE',  ( -14.47279130897152299, 14.42499999726880056, 19.92008829642072243 ) ) ;
#5700=CARTESIAN_POINT ( 'NONE',  ( -14.47279130897152122, 7.924999997268803220, 19.92008829642072243 ) ) ;
#5722=CARTESIAN_POINT ( 'NONE',  ( -23.41746825000000598, 13.72499999726882258, 7.608796670333726198 ) ) ;
#5723=CARTESIAN_POINT ( 'NONE',  ( 0.000000000000000000, 16.99999999999998579, 0.000000000000000000 ) ) ;
#5746=CARTESIAN_POINT ( 'NONE',  ( -15.14183272437241889, 16.44999999453761319, -20.84094480462497856 ) ) ;
#5755=DIRECTION ( 'NONE',  ( 0.000000000000000000, -1.000000000000000000, 0.000000000000000000 ) ) ;
#5759=CARTESIAN_POINT ( 'NONE',  ( 18.94512977948575738, 12.92499999726881654, 13.76444248337723408 ) ) ;
#5783=CARTESIAN_POINT ( 'NONE',  ( -3.880418787951174675, 10.55125428154683931, -24.49999999999998579 ) ) ;
#5790=CARTESIAN_POINT ( 'NONE',  ( 0.000000000000000000, 16.99999999999998579, 0.000000000000000000 ) ) ;
#5824=CARTESIAN_POINT ( 'NONE',  ( -24.50000000000000355, 8.900000000000011013, -7.960532557706207157 ) ) ;
#5826=CARTESIAN_POINT ( 'NONE',  ( -19.82091636218621034, 6.549999994537619941, -14.40073868116559552 ) ) ;
#5829=CARTESIAN_POINT ( 'NONE',  ( 18.94512977948576093, 6.824999997268821339, -13.76444248337722875 ) ) ;
#5833=CARTESIAN_POINT ( 'NONE',  ( 22.22281446566211116, 16.99999999999998224, -7.541208221400177436 ) ) ;
#5847=CARTESIAN_POINT ( 'NONE',  ( 23.41746824999999887, 15.02499999726881086, 7.608796670333735079 ) ) ;
#5863=CARTESIAN_POINT ( 'NONE',  ( -4.523095164977116484E-15, 6.124999997268802510, 24.62258325217400312 ) ) ;
#5871=CARTESIAN_POINT ( 'NONE',  ( 7.236395654485755280, 16.72499999726881370, 22.27133577429736988 ) ) ;
#5886=CARTESIAN_POINT ( 'NONE',  ( 7.236395654485760609, 17.02499999726880731, -22.27133577429736633 ) ) ;
#5897=CARTESIAN_POINT ( 'NONE',  ( -24.50000000000000711, 2.849999994537638859, 7.960532557706201828 ) ) ;
#5901=VECTOR ( 'NONE', #855, 1000.000000000000000 ) ;
#5912=CARTESIAN_POINT ( 'NONE',  ( -23.41746825000000598, 2.224999997268808816, 7.608796670333726198 ) ) ;
#5927=CARTESIAN_POINT ( 'NONE',  ( -23.41746825000000598, 12.22499999726881370, 7.608796670333726198 ) ) ;
#5957=DIRECTION ( 'NONE',  ( 0.000000000000000000, 0.000000000000000000, -1.000000000000000000 ) ) ;
#5959=CARTESIAN_POINT ( 'NONE',  ( 0.000000000000000000, 16.99999999999998579, -24.50000000000000000 ) ) ;
#5968=CARTESIAN_POINT ( 'NONE',  ( -24.50000000000000000, 13.00000000000001066, -3.000384657911015469E-15 ) ) ;
#5987=CARTESIAN_POINT ( 'NONE',  ( 1.577395562988744260E-15, 14.50000000000000888, -25.76082449383753925 ) ) ;
#5990=CARTESIAN_POINT ( 'NONE',  ( -4.523095164977117273E-15, 10.12499999726882116, 24.62258325217400312 ) ) ;
#5995=CARTESIAN_POINT ( 'NONE',  ( 23.41787895562451638, 16.99999999999998224, 0.7516208871782403822 ) ) ;
#6020=CARTESIAN_POINT ( 'NONE',  ( 3.880418787951140036, 12.44874571845315714, -24.49999999999999645 ) ) ;
#6023=CARTESIAN_POINT ( 'NONE',  ( 7.236395654485760609, 11.02499999726880375, -22.27133577429736633 ) ) ;
#6042=CARTESIAN_POINT ( 'NONE',  ( -23.41746825000000598, 15.72499999726882081, 7.608796670333726198 ) ) ;
#6053=CARTESIAN_POINT ( 'NONE',  ( -24.50000000000000000, 2.649999994537616477, -7.960532557706207157 ) ) ;
#6067=CARTESIAN_POINT ( 'NONE',  ( -23.41746825000000243, 2.024999997268815299, -7.608796670333730638 ) ) ;
#6085=CARTESIAN_POINT ( 'NONE',  ( -23.41746825000000243, 16.02499999726881086, -7.608796670333730638 ) ) ;
#6105=CARTESIAN_POINT ( 'NONE',  ( -4.223320258572819786E-15, 9.499999999999992895, 24.50000000000000000 ) ) ;
#6110=DIRECTION ( 'NONE',  ( 0.000000000000000000, -1.000000000000000000, 0.000000000000000000 ) ) ;
#6135=CARTESIAN_POINT ( 'NONE',  ( 24.50000000000000000, 15.74999999453763344, 0.000000000000000000 ) ) ;
#6136=APPLICATION_CONTEXT ( 'automotive_design' ) ;
#6147=CARTESIAN_POINT ( 'NONE',  ( -19.82091636218621034, 8.800000000000002487, -14.40073868116559552 ) ) ;
#6152=CARTESIAN_POINT ( 'NONE',  ( 7.236395654485760609, 11.02499999726880375, -22.27133577429736633 ) ) ;
#6174=DIRECTION ( 'NONE',  ( 0.000000000000000000, 0.000000000000000000, -1.000000000000000000 ) ) ;
#6184=CARTESIAN_POINT ( 'NONE',  ( 24.50000000000000000, 12.00000000000001066, 0.000000000000000000 ) ) ;
#6186=CARTESIAN_POINT ( 'NONE',  ( 0.000000000000000000, 0.000000000000000000, 0.000000000000000000 ) ) ;
#6188=CARTESIAN_POINT ( 'NONE',  ( 1.507698388325705758E-15, 11.12499999726881761, -24.62258325217400312 ) ) ;
#6195=AXIS2_PLACEMENT_3D ( 'NONE', #6607, #11753, #9516 ) ;
#6210=CARTESIAN_POINT ( 'NONE',  ( 23.41746825000000243, 16.72499999726881725, -7.608796670333727974 ) ) ;
#6215=CARTESIAN_POINT ( 'NONE',  ( 1.507698388325705758E-15, 1.624999997268827823, -24.62258325217400312 ) ) ;
#6239=CARTESIAN_POINT ( 'NONE',  ( -14.47279130897151589, 5.824999997268811569, -19.92008829642072598 ) ) ;
#6256=CARTESIAN_POINT ( 'NONE',  ( -4.523095164977116484E-15, 12.62499999726879985, 24.62258325217400312 ) ) ;
#6265=CARTESIAN_POINT ( 'NONE',  ( 6.001560367445586717E-15, 1.500000000000005995, 24.50000000000000000 ) ) ;
#6266=VERTEX_POINT ( 'NONE', #25981 ) ;
#6281=CARTESIAN_POINT ( 'NONE',  ( -24.50000000000000711, 16.84999999453763309, 7.960532557706201828 ) ) ;
#6288=CARTESIAN_POINT ( 'NONE',  ( 19.42321331973577969, 16.99999999999997868, 13.32227027544421638 ) ) ;
#6296=CARTESIAN_POINT ( 'NONE',  ( -24.50000000000000711, 10.84999999453761887, 7.960532557706201828 ) ) ;
#6325=CARTESIAN_POINT ( 'NONE',  ( 1.577395562988744260E-15, 12.50000000000001243, -25.76082449383753925 ) ) ;
#6329=CARTESIAN_POINT ( 'NONE',  ( -23.41746824999999887, 9.624999997268817609, -2.867812753649727150E-15 ) ) ;
#6330=CARTESIAN_POINT ( 'NONE',  ( 24.50000000000000000, 3.649999994537613812, 7.960532557706212486 ) ) ;
#6333=CARTESIAN_POINT ( 'NONE',  ( 19.90391271886689495, 16.99999999999998579, -12.36117064040718461 ) ) ;
#6337=CARTESIAN_POINT ( 'NONE',  ( 0.000000000000000000, 16.99999999999998579, 0.000000000000000000 ) ) ;
#6343=EDGE_LOOP ( 'NONE', ( #17736, #26529, #28727, #8040 ) ) ;
#6361=CARTESIAN_POINT ( 'NONE',  ( 14.47279130897151589, 14.32499999726880624, 19.92008829642072953 ) ) ;
#6391=VERTEX_POINT ( 'NONE', #3318 ) ;
#6397=DIRECTION ( 'NONE',  ( 0.000000000000000000, 0.000000000000000000, -1.000000000000000000 ) ) ;
#6412=CARTESIAN_POINT ( 'NONE',  ( -23.41746825000000598, 8.224999997268824359, 7.608796670333726198 ) ) ;
#6423=CARTESIAN_POINT ( 'NONE',  ( 3.880418787951102289, 16.44874571845315359, -24.50000000000000711 ) ) ;
#6427=CARTESIAN_POINT ( 'NONE',  ( 23.41746824999999887, 4.624999997268814056, 0.000000000000000000 ) ) ;
#6451=CARTESIAN_POINT ( 'NONE',  ( 0.000000000000000000, 16.99999999999998579, 0.000000000000000000 ) ) ;
#6452=CARTESIAN_POINT ( 'NONE',  ( 7.570916362186207671, 5.349999994537641079, 23.30088464923126779 ) ) ;
#6459=CARTESIAN_POINT ( 'NONE',  ( 0.5672726147806251840, 16.99999999999999289, 24.06736868777154470 ) ) ;
#6463=DIRECTION ( 'NONE',  ( 0.000000000000000000, -1.000000000000000000, 0.000000000000000000 ) ) ;
#6468=DIRECTION ( 'NONE',  ( 0.000000000000000000, 0.000000000000000000, -1.000000000000000000 ) ) ;
#6470=CARTESIAN_POINT ( 'NONE',  ( -7.570916362186210335, 12.59999999999999964, -23.30088464923126779 ) ) ;
#6481=CARTESIAN_POINT ( 'NONE',  ( 15.14183272437242422, 16.04999999453762882, -20.84094480462497856 ) ) ;
#6494=CARTESIAN_POINT ( 'NONE',  ( -24.50000000000001066, 13.09999999999999432, 7.960532557706201828 ) ) ;
#6498=CARTESIAN_POINT ( 'NONE',  ( -23.41746824999999887, 7.624999997268816720, -2.867812753649727150E-15 ) ) ;
#6515=EDGE_CURVE ( 'NONE', #22342, #16741, #2810, .T. ) ;
#6533=CARTESIAN_POINT ( 'NONE',  ( 7.236395654485760609, 9.024999997268828622, -22.27133577429736633 ) ) ;
#6539=ORIENTED_EDGE ( 'NONE', *, *, #16824, .F. ) ;
#6559=VERTEX_POINT ( 'NONE', #13950 ) ;
#6577=CARTESIAN_POINT ( 'NONE',  ( -23.41746825000000243, 8.024999997268801977, -7.608796670333730638 ) ) ;
#6588=CARTESIAN_POINT ( 'NONE',  ( 24.50000000000000000, 7.649999994537632908, 7.960532557706212486 ) ) ;
#6590=CARTESIAN_POINT ( 'NONE',  ( -14.47279130897151589, 5.324999997268826668, -19.92008829642072598 ) ) ;
#6596=PRODUCT_DEFINITION_FORMATION_WITH_SPECIFIED_SOURCE ( 'ANY', '', #32094, .NOT_KNOWN. ) ;
#6597=EDGE_LOOP ( 'NONE', ( #8292, #17548 ) ) ;
#6607=CARTESIAN_POINT ( 'NONE',  ( 0.000000000000000000, 16.99999999999998579, 0.000000000000000000 ) ) ;
#6614=CARTESIAN_POINT ( 'NONE',  ( -7.570916362186215665, 5.149999994537635573, 23.30088464923126423 ) ) ;
#6628=CARTESIAN_POINT ( 'NONE',  ( -23.41746825000000243, 4.024999997268810858, -7.608796670333730638 ) ) ;
#6656=CARTESIAN_POINT ( 'NONE',  ( 24.50000000000000355, 16.09999999999998366, -7.960532557706203605 ) ) ;
#6661=CARTESIAN_POINT ( 'NONE',  ( -14.47279130897152299, 7.924999997268802332, 19.92008829642072243 ) ) ;
#6693=CARTESIAN_POINT ( 'NONE',  ( 18.94512977948575738, 8.424999997268811214, 13.76444248337723408 ) ) ;
#6719=CARTESIAN_POINT ( 'NONE',  ( -23.41746824999999887, 4.124999997268813168, -2.867812753649727150E-15 ) ) ;
#6732=EDGE_CURVE ( 'NONE', #19356, #16549, #16993, .T. ) ;
#6738=CARTESIAN_POINT ( 'NONE',  ( 15.14183272437242422, 8.300000000000000711, -20.84094480462497856 ) ) ;
#6743=CARTESIAN_POINT ( 'NONE',  ( 14.47279130897151767, 9.424999997268814766, -19.92008829642072598 ) ) ;
#6757=CARTESIAN_POINT ( 'NONE',  ( -7.236395654485757944, 3.224999997268801266, -22.27133577429736988 ) ) ;
#6760=( BOUNDED_CURVE ( )  B_SPLINE_CURVE ( 2, ( #1648, #30650, #25169, #12642, #9553, #4920, #25001, #9724, #30478, #33403, #30826, #4405, #20032 ),
 .UNSPECIFIED., .F., .T. ) 
 B_SPLINE_CURVE_WITH_KNOTS ( ( 3, 2, 2, 2, 2, 2, 3 ),
 ( 0.3611111111111111049, 0.3666666666666666408, 0.3777777777777777679, 0.3888888888888888951, 0.4000000000000000222, 0.4111111111111110938, 0.4166666666666666852 ),
 .UNSPECIFIED. ) 
 CURVE ( )  GEOMETRIC_REPRESENTATION_ITEM ( )  RATIONAL_B_SPLINE_CURVE ( ( 0.9755282581475768211, 0.9755282581475768211, 1.000000000000000000, 0.9510565162951535312, 1.000000000000000000, 0.9510565162951535312, 1.000000000000000000, 0.9510565162951535312, 1.000000000000000000, 0.9510565162951535312, 1.000000000000000000, 0.9755282581475765991, 0.9755282581475767101 ) ) 
 REPRESENTATION_ITEM ( '' )  );
#6782=CARTESIAN_POINT ( 'NONE',  ( 7.570916362186213000, 8.149999994537637349, -23.30088464923126423 ) ) ;
#6791=CARTESIAN_POINT ( 'NONE',  ( 7.570916362186207671, 1.599999999999990319, 23.30088464923126779 ) ) ;
#6795=CARTESIAN_POINT ( 'NONE',  ( -18.94512977948575738, 3.924999997268807661, -13.76444248337723231 ) ) ;
#6797=FACE_OUTER_BOUND ( 'NONE', #33883, .T. ) ;
#6807=CARTESIAN_POINT ( 'NONE',  ( -24.50000000000000711, 3.099999999999989431, 7.960532557706201828 ) ) ;
#6825=CARTESIAN_POINT ( 'NONE',  ( 14.47279130897151767, 14.32499999726880624, 19.92008829642072953 ) ) ;
#6830=CARTESIAN_POINT ( 'NONE',  ( -6.391981326054763102, 16.99999999999998224, -22.99215804002973940 ) ) ;
#6837=ADVANCED_FACE ( 'NONE', ( #8747 ), #24377, .T. ) ;
#6840=LINE ( 'NONE', #28122, #3022 ) ;
#6864=CARTESIAN_POINT ( 'NONE',  ( 7.570916362186207671, 1.599999999999990319, 23.30088464923126779 ) ) ;
#6903=CARTESIAN_POINT ( 'NONE',  ( -23.41746825000000243, 1.524999997268801755, -7.608796670333730638 ) ) ;
#6913=CARTESIAN_POINT ( 'NONE',  ( 18.94512977948576093, 7.324999997268822227, -13.76444248337722875 ) ) ;
#6925=CARTESIAN_POINT ( 'NONE',  ( -7.236395654485757944, 1.224999997268799712, -22.27133577429736988 ) ) ;
#6950=CARTESIAN_POINT ( 'NONE',  ( -19.82091636218621389, 4.949999994537629178, 14.40073868116558842 ) ) ;
#6958=DIRECTION ( 'NONE',  ( 0.000000000000000000, 0.000000000000000000, -1.000000000000000000 ) ) ;
#6965=CARTESIAN_POINT ( 'NONE',  ( 14.47279130897151589, 4.824999997268814234, 19.92008829642072953 ) ) ;
#6967=CYLINDRICAL_SURFACE ( 'NONE', #15649, 24.50000000000000000 ) ;
#6991=AXIS2_PLACEMENT_3D ( 'NONE', #29401, #21525, #24753 ) ;
#6994=CARTESIAN_POINT ( 'NONE',  ( -7.570916362186215665, 15.39999999999999680, 23.30088464923126423 ) ) ;
#6999=CARTESIAN_POINT ( 'NONE',  ( 18.94512977948575738, 14.42499999726881654, 13.76444248337723408 ) ) ;
#7028=CARTESIAN_POINT ( 'NONE',  ( 7.313012447739250820E-14, 13.24999999453762456, 24.50000000000000000 ) ) ;
#7032=CARTESIAN_POINT ( 'NONE',  ( 18.94512977948575738, 16.42499999726882010, 13.76444248337723408 ) ) ;
#7048=CARTESIAN_POINT ( 'NONE',  ( 24.50000000000000000, 15.89999999999998970, 7.960532557706212486 ) ) ;
#7057=( BOUNDED_CURVE ( )  B_SPLINE_CURVE ( 2, ( #8421, #16836, #8592, #3783, #9094, #32265, #6184, #14254, #11670, #22151, #19576, #6020, #30024 ),
 .UNSPECIFIED., .F., .T. ) 
 B_SPLINE_CURVE_WITH_KNOTS ( ( 3, 2, 2, 2, 2, 2, 3 ),
 ( 0.6388888888888889506, 0.6444444444444444864, 0.6555555555555555580, 0.6666666666666666297, 0.6777777777777778123, 0.6888888888888888840, 0.6944444444444444198 ),
 .UNSPECIFIED. ) 
 CURVE ( )  GEOMETRIC_REPRESENTATION_ITEM ( )  RATIONAL_B_SPLINE_CURVE ( ( 0.9755282581475768211, 0.9755282581475770431, 1.000000000000000000, 0.9510565162951535312, 1.000000000000000000, 0.9510565162951535312, 1.000000000000000000, 0.9510565162951535312, 1.000000000000000000, 0.9510565162951535312, 1.000000000000000000, 0.9755282581475768211, 0.9755282581475768211 ) ) 
 REPRESENTATION_ITEM ( '' )  );
#7058=CARTESIAN_POINT ( 'NONE',  ( -14.47279130897152299, 10.42499999726881121, 19.92008829642072243 ) ) ;
#7082=CARTESIAN_POINT ( 'NONE',  ( -23.41746824999999887, 16.12499999726882294, -2.867812753649727150E-15 ) ) ;
#7095=CARTESIAN_POINT ( 'NONE',  ( 1.507698388325705758E-15, 3.124999997268809615, -24.62258325217400312 ) ) ;
#7103=ORIENTED_EDGE ( 'NONE', *, *, #5280, .T. ) ;
#7119=CARTESIAN_POINT ( 'NONE',  ( 19.82091636218621034, 11.54999999453762349, 14.40073868116559730 ) ) ;
#7134=CARTESIAN_POINT ( 'NONE',  ( 18.94512977948575738, 2.924999997268806773, 13.76444248337723408 ) ) ;
#7162=CARTESIAN_POINT ( 'NONE',  ( 24.50000000000000355, 15.89999999999999147, 7.960532557706212486 ) ) ;
#7168=CARTESIAN_POINT ( 'NONE',  ( 14.47279130897151767, 16.32499999726882933, 19.92008829642072953 ) ) ;
#7172=CARTESIAN_POINT ( 'NONE',  ( -3.880418787951146697, 4.301254276084477191, -24.49999999999999645 ) ) ;
#7173=DIRECTION ( 'NONE',  ( 0.000000000000000000, -1.000000000000000000, 0.000000000000000000 ) ) ;
#7203=CARTESIAN_POINT ( 'NONE',  ( -14.47279130897151589, 17.32499999726879381, -19.92008829642072598 ) ) ;
#7205=PLANE ( 'NONE',  #30991 ) ;
#7227=CARTESIAN_POINT ( 'NONE',  ( 18.94512977948575738, 10.92499999726881299, 13.76444248337723408 ) ) ;
#7250=CARTESIAN_POINT ( 'NONE',  ( -4.523095164977116484E-15, 16.62499999726881583, 24.62258325217400312 ) ) ;
#7251=CARTESIAN_POINT ( 'NONE',  ( -23.41746825000000243, 5.724999997268815477, 7.608796670333725309 ) ) ;
#7265=CARTESIAN_POINT ( 'NONE',  ( 23.41746824999999887, 8.624999997268817609, 0.000000000000000000 ) ) ;
#7272=AXIS2_PLACEMENT_3D ( 'NONE', #23015, #21128, #7390 ) ;
#7291=CARTESIAN_POINT ( 'NONE',  ( 24.50000000000000355, 15.64999999453761426, 7.960532557706212486 ) ) ;
#7305=CARTESIAN_POINT ( 'NONE',  ( 7.236395654485760609, 3.524999997268824181, -22.27133577429736633 ) ) ;
#7317=CARTESIAN_POINT ( 'NONE',  ( 7.570916362186213000, 10.39999999999999325, -23.30088464923126423 ) ) ;
#7326=CARTESIAN_POINT ( 'NONE',  ( -24.50000000000000000, 4.899999999999990585, -7.960532557706207157 ) ) ;
#7335=CARTESIAN_POINT ( 'NONE',  ( -4.732186688966233175E-15, 17.50000000000000000, 25.76082449383753925 ) ) ;
#7340=CARTESIAN_POINT ( 'NONE',  ( 15.07600611976209848, 16.91151231482331596, -19.08983433668813134 ) ) ;
#7343=CARTESIAN_POINT ( 'NONE',  ( -14.34159108954266770, 16.99999999999999289, -19.25229178662170071 ) ) ;
#7347=CARTESIAN_POINT ( 'NONE',  ( -3.880418787951104953, 13.19874571299077459, 24.50000000000000711 ) ) ;
#7349=DIRECTION ( 'NONE',  ( -0.000000000000000000, 1.000000000000000000, -0.000000000000000000 ) ) ;
#7374=CARTESIAN_POINT ( 'NONE',  ( 24.50000000000000000, 13.84999999453761177, -7.960532557706203605 ) ) ;
#7379=CARTESIAN_POINT ( 'NONE',  ( 1.577395562988744260E-15, 0.5000000000000133227, -25.76082449383753925 ) ) ;
#7390=DIRECTION ( 'NONE',  ( 1.000000000000000000, 0.000000000000000000, -0.000000000000000000 ) ) ;
#7393=CARTESIAN_POINT ( 'NONE',  ( 24.50000000000000000, 15.99999999999998579, 0.000000000000000000 ) ) ;
#7404=CARTESIAN_POINT ( 'NONE',  ( 18.94512977948575738, 8.924999997268812990, 13.76444248337723408 ) ) ;
#7429=CARTESIAN_POINT ( 'NONE',  ( 1.507698388325705758E-15, 13.62499999726882827, -24.62258325217400312 ) ) ;
#7430=CARTESIAN_POINT ( 'NONE',  ( 18.94512977948576093, 2.824999997268817786, -13.76444248337722875 ) ) ;
#7438=UNCERTAINTY_MEASURE_WITH_UNIT (LENGTH_MEASURE( 1.000000000000000082E-05 ), #12529, 'distance_accuracy_value', 'NONE');
#7446=CARTESIAN_POINT ( 'NONE',  ( -14.47279130897151589, 7.324999997268822227, -19.92008829642072598 ) ) ;
#7447=CARTESIAN_POINT ( 'NONE',  ( 7.570916362186207671, 13.60000000000000142, 23.30088464923126779 ) ) ;
#7454=APPLICATION_CONTEXT ( 'automotive_design' ) ;
#7471=ADVANCED_FACE ( 'NONE', ( #10752 ), #33270, .T. ) ;
#7473=CARTESIAN_POINT ( 'NONE',  ( -4.732186688966233175E-15, 11.24999999453763699, 25.76082449383753925 ) ) ;
#7482=EDGE_CURVE ( 'NONE', #31792, #24787, #18488, .T. ) ;
#7488=CARTESIAN_POINT ( 'NONE',  ( 14.47279130897151767, 11.42499999726880944, -19.92008829642072598 ) ) ;
#7552=CARTESIAN_POINT ( 'NONE',  ( -7.570916362186210335, 0.5999999999999894307, -23.30088464923126779 ) ) ;
#7566=CARTESIAN_POINT ( 'NONE',  ( 7.570916362186213000, 6.399999999999988809, -23.30088464923126423 ) ) ;
#7578=CARTESIAN_POINT ( 'NONE',  ( 18.94512977948575738, 4.924999997268808549, 13.76444248337723408 ) ) ;
#7601=EDGE_LOOP ( 'NONE', ( #10702, #30997, #10575, #15483 ) ) ;
#7602=CARTESIAN_POINT ( 'NONE',  ( -7.236395654485757944, 11.72499999726880837, -22.27133577429736988 ) ) ;
#7603=CARTESIAN_POINT ( 'NONE',  ( 1.507698388325705758E-15, 3.124999997268809615, -24.62258325217400312 ) ) ;
#7615=CARTESIAN_POINT ( 'NONE',  ( 7.236395654485755280, 10.22499999726880837, 22.27133577429736988 ) ) ;
#7639=CARTESIAN_POINT ( 'NONE',  ( 24.50000000000000000, 11.74999999453762989, 0.000000000000000000 ) ) ;
#7647=CARTESIAN_POINT ( 'NONE',  ( -15.14183272437242067, 6.699999999999991296, -20.84094480462497856 ) ) ;
#7653=CARTESIAN_POINT ( 'NONE',  ( -14.47279130897151589, 11.82499999726882578, -19.92008829642072598 ) ) ;
#7669=( BOUNDED_CURVE ( )  B_SPLINE_CURVE ( 2, ( #18724, #11315, #8900, #3590, #13897, #8230, #21626 ),
 .UNSPECIFIED., .F., .T. ) 
 B_SPLINE_CURVE_WITH_KNOTS ( ( 3, 2, 2, 3 ),
 ( 0.000000000000000000, 0.01111111111111111154, 0.02222222222222222307, 0.02777777777777777971 ),
 .UNSPECIFIED. ) 
 CURVE ( )  GEOMETRIC_REPRESENTATION_ITEM ( )  RATIONAL_B_SPLINE_CURVE ( ( 1.000000000000000000, 0.9510565162951535312, 1.000000000000000000, 0.9510565162951535312, 1.000000000000000000, 0.9755282581475768211, 0.9755282581475768211 ) ) 
 REPRESENTATION_ITEM ( '' )  );
#7693=CARTESIAN_POINT ( 'NONE',  ( -7.570916362186215665, 13.14999999453761426, 23.30088464923126423 ) ) ;
#7694=CARTESIAN_POINT ( 'NONE',  ( 0.000000000000000000, -20.99999999999998934, -24.50000000000000000 ) ) ;
#7720=CARTESIAN_POINT ( 'NONE',  ( 24.50000000000000000, 8.000000000000007105, 0.000000000000000000 ) ) ;
#7722=CARTESIAN_POINT ( 'NONE',  ( 24.50000000000000355, 1.849999994537612436, -7.960532557706203605 ) ) ;
#7742=CARTESIAN_POINT ( 'NONE',  ( -23.41746825000000243, 10.22499999726881725, 7.608796670333725309 ) ) ;
#7761=CARTESIAN_POINT ( 'NONE',  ( -14.47279130897152122, 5.924999997268808549, 19.92008829642072243 ) ) ;
#7770=CARTESIAN_POINT ( 'NONE',  ( 7.236395654485755280, 14.72499999726881192, 22.27133577429736988 ) ) ;
#7782=CARTESIAN_POINT ( 'NONE',  ( -18.94512977948576093, 9.824999997268824004, 13.76444248337722698 ) ) ;
#7807=CARTESIAN_POINT ( 'NONE',  ( 24.50000000000000355, 11.64999999453762314, 7.960532557706212486 ) ) ;
#7818=VECTOR ( 'NONE', #1335, 1000.000000000000114 ) ;
#7823=CARTESIAN_POINT ( 'NONE',  ( -18.94512977948575738, 7.924999997268811214, -13.76444248337723231 ) ) ;
#7832=CARTESIAN_POINT ( 'NONE',  ( 24.50000000000000000, 10.10000000000000142, -7.960532557706203605 ) ) ;
#7860=CARTESIAN_POINT ( 'NONE',  ( -7.570916362186210335, 12.34999999453761887, -23.30088464923126779 ) ) ;
#7867=EDGE_LOOP ( 'NONE', ( #26364, #32979 ) ) ;
#7884=EDGE_CURVE ( 'NONE', #9893, #24093, #27312, .T. ) ;
#7887=CARTESIAN_POINT ( 'NONE',  ( -24.50000000000000355, 6.900000000000014566, -7.960532557706207157 ) ) ;
#7889=CARTESIAN_POINT ( 'NONE',  ( -24.50000000000001066, 2.849999994537639303, 7.960532557706201828 ) ) ;
#7914=CARTESIAN_POINT ( 'NONE',  ( -23.41746824999999887, 14.02499999726881263, -7.608796670333730638 ) ) ;
#7930=CARTESIAN_POINT ( 'NONE',  ( 7.236395654485760609, 7.024999997268826846, -22.27133577429736633 ) ) ;
#7953=CARTESIAN_POINT ( 'NONE',  ( -7.236395654485757944, 11.22499999726880837, -22.27133577429736988 ) ) ;
#7954=CARTESIAN_POINT ( 'NONE',  ( -4.223320258572819786E-15, 3.499999999999996891, 24.50000000000000000 ) ) ;
#7977=CARTESIAN_POINT ( 'NONE',  ( -14.47279130897151589, 1.824999997268821339, -19.92008829642072598 ) ) ;
#7984=CARTESIAN_POINT ( 'NONE',  ( 1.555960095263670572E-15, 6.499999999999994671, -24.50000000000000000 ) ) ;
#7994=CARTESIAN_POINT ( 'NONE',  ( 18.94512977948576093, 7.324999997268822227, -13.76444248337722875 ) ) ;
#8004=EDGE_LOOP ( 'NONE', ( #27492, #23500, #28300, #4322, #32708, #32999, #17114, #25849, #17588, #2038, #14746, #20765, #14705, #25472, #4318, #20484, #27329, #15784, #9811, #31943, #14328 ) ) ;
#8006=LINE ( 'NONE', #18660, #18812 ) ;
#8040=ORIENTED_EDGE ( 'NONE', *, *, #16915, .T. ) ;
#8058=CARTESIAN_POINT ( 'NONE',  ( 24.50000000000000000, 6.000000000000005329, 0.000000000000000000 ) ) ;
#8083=CARTESIAN_POINT ( 'NONE',  ( -14.47279130897151767, 15.82499999726881512, -19.92008829642072598 ) ) ;
#8099=CARTESIAN_POINT ( 'NONE',  ( 18.94512977948576093, 6.824999997268821339, -13.76444248337722875 ) ) ;
#8107=ORIENTED_EDGE ( 'NONE', *, *, #19434, .F. ) ;
#8121=CARTESIAN_POINT ( 'NONE',  ( 18.94512977948575738, 18.42499999726882010, 13.76444248337723408 ) ) ;
#8147=CARTESIAN_POINT ( 'NONE',  ( 23.41746824999999887, 3.124999997268812280, 0.000000000000000000 ) ) ;
#8159=CARTESIAN_POINT ( 'NONE',  ( 23.41746825000000243, 7.024999997268802865, 7.608796670333735079 ) ) ;
#8194=CARTESIAN_POINT ( 'NONE',  ( 19.82091636218621034, 11.54999999453762349, 14.40073868116559730 ) ) ;
#8220=CARTESIAN_POINT ( 'NONE',  ( 1.577395562988744260E-15, 2.500000000000008882, -25.76082449383753925 ) ) ;
#8225=CARTESIAN_POINT ( 'NONE',  ( 23.41746824999999887, 6.524999997268818852, 7.608796670333735079 ) ) ;
#8226=CARTESIAN_POINT ( 'NONE',  ( -24.50000000000000000, 8.900000000000011013, -7.960532557706207157 ) ) ;
#8229=CARTESIAN_POINT ( 'NONE',  ( 19.82091636218621034, 9.549999994537621717, 14.40073868116559730 ) ) ;
#8230=CARTESIAN_POINT ( 'NONE',  ( 3.880418787951139148, 2.198745712990784806, -24.50000000000000000 ) ) ;
#8233=CYLINDRICAL_SURFACE ( 'NONE', #33050, 24.50000000000000000 ) ;
#8243=CARTESIAN_POINT ( 'NONE',  ( 18.94512977948576093, 13.32499999726879913, -13.76444248337722875 ) ) ;
#8260=CARTESIAN_POINT ( 'NONE',  ( 18.94512977948575738, 4.424999997268807661, 13.76444248337723408 ) ) ;
#8267=EDGE_LOOP ( 'NONE', ( #4639, #15658, #7103, #21992 ) ) ;
#8268=CARTESIAN_POINT ( 'NONE',  ( -14.47279130897151589, 17.82499999726881157, -19.92008829642072598 ) ) ;
#8280=CARTESIAN_POINT ( 'NONE',  ( 18.94512977948575738, 14.42499999726881654, 13.76444248337723408 ) ) ;
#8292=ORIENTED_EDGE ( 'NONE', *, *, #13074, .T. ) ;
#8293=CARTESIAN_POINT ( 'NONE',  ( -15.14183272437242067, 2.449999994537622960, -20.84094480462497856 ) ) ;
#8307=CARTESIAN_POINT ( 'NONE',  ( -24.50000000000000000, 18.74999999453763522, -3.000384657911015469E-15 ) ) ;
#8323=CARTESIAN_POINT ( 'NONE',  ( -14.47279130897151589, 17.82499999726881157, -19.92008829642072598 ) ) ;
#8325=ORIENTED_EDGE ( 'NONE', *, *, #6515, .T. ) ;
#8355=DIRECTION ( 'NONE',  ( 0.000000000000000000, -1.000000000000000000, 0.000000000000000000 ) ) ;
#8363=CARTESIAN_POINT ( 'NONE',  ( -7.570916362186215665, 11.14999999453761248, 23.30088464923126423 ) ) ;
#8388=CARTESIAN_POINT ( 'NONE',  ( 7.570916362186207671, 5.599999999999994316, 23.30088464923126779 ) ) ;
#8393=CARTESIAN_POINT ( 'NONE',  ( 7.236395654485755280, 6.224999997268803931, 22.27133577429736988 ) ) ;
#8396=CARTESIAN_POINT ( 'NONE',  ( 17.62835169016977233, 16.99999999999998579, -15.43382168286624179 ) ) ;
#8411=CARTESIAN_POINT ( 'NONE',  ( -7.236395654485763274, 12.52499999726880375, 22.27133577429736633 ) ) ;
#8421=CARTESIAN_POINT ( 'NONE',  ( 7.313012447739250820E-14, 11.49999999999999112, 24.50000000000000000 ) ) ;
#8428=CARTESIAN_POINT ( 'NONE',  ( -14.47279130897151589, 3.324999997268803131, -19.92008829642072598 ) ) ;
#8450=CARTESIAN_POINT ( 'NONE',  ( 1.507698388325705758E-15, 17.12499999726880517, -24.62258325217400312 ) ) ;
#8452=CARTESIAN_POINT ( 'NONE',  ( 24.50000000000000000, 13.89999999999999680, 7.960532557706212486 ) ) ;
#8463=CARTESIAN_POINT ( 'NONE',  ( -3.880418787951138260, 3.198745712990784806, 24.50000000000000000 ) ) ;
#8479=CARTESIAN_POINT ( 'NONE',  ( 14.47279130897151767, 1.424999997268804997, -19.92008829642072598 ) ) ;
#8493=CARTESIAN_POINT ( 'NONE',  ( 7.236395654485755280, 14.72499999726881192, 22.27133577429736988 ) ) ;
#8514=LINE ( 'NONE', #11103, #21461 ) ;
#8527=CARTESIAN_POINT ( 'NONE',  ( -5.260389231090357498, 16.99999999999999289, 23.61507992718642868 ) ) ;
#8529=CARTESIAN_POINT ( 'NONE',  ( 15.14183272437242422, 12.04999999453761106, -20.84094480462497856 ) ) ;
#8561=CARTESIAN_POINT ( 'NONE',  ( 19.82091636218621034, 11.80000000000000426, 14.40073868116559730 ) ) ;
#8564=CARTESIAN_POINT ( 'NONE',  ( -4.523095164977117273E-15, 12.12499999726881583, 24.62258325217400312 ) ) ;
#8582=CARTESIAN_POINT ( 'NONE',  ( 23.41746824999999887, 15.22499999726880482, -7.608796670333727974 ) ) ;
#8592=CARTESIAN_POINT ( 'NONE',  ( 7.570916362186207671, 11.59999999999999964, 23.30088464923126779 ) ) ;
#8596=CARTESIAN_POINT ( 'NONE',  ( -7.236395654485763274, 12.02499999726880375, 22.27133577429736633 ) ) ;
#8607=CYLINDRICAL_SURFACE ( 'NONE', #2542, 24.50000000000000000 ) ;
#8615=AXIS2_PLACEMENT_3D ( 'NONE', #31048, #10965, #21439 ) ;
#8620=CARTESIAN_POINT ( 'NONE',  ( 14.47279130897151767, 14.92499999726881299, -19.92008829642072598 ) ) ;
#8644=CARTESIAN_POINT ( 'NONE',  ( 1.507698388325705758E-15, 3.624999997268822938, -24.62258325217400312 ) ) ;
#8660=CARTESIAN_POINT ( 'NONE',  ( 14.47279130897151589, 14.82499999726881690, 19.92008829642072953 ) ) ;
#8693=CARTESIAN_POINT ( 'NONE',  ( -6.220434760165790777, 16.99999999999999645, 23.40342332511181667 ) ) ;
#8723=CARTESIAN_POINT ( 'NONE',  ( -7.570916362186215665, 9.399999999999991473, 23.30088464923126423 ) ) ;
#8728=CARTESIAN_POINT ( 'NONE',  ( -23.41746824999999887, 7.524999997268816188, -7.608796670333730638 ) ) ;
#8730=CARTESIAN_POINT ( 'NONE',  ( 15.14183272437242422, 4.300000000000009592, -20.84094480462497856 ) ) ;
#8747=FACE_OUTER_BOUND ( 'NONE', #29426, .T. ) ;
#8761=CARTESIAN_POINT ( 'NONE',  ( 18.94512977948576093, 10.82499999726882578, -13.76444248337722875 ) ) ;
#8781=CARTESIAN_POINT ( 'NONE',  ( -23.41746824999999887, 15.62499999726882294, -2.867812753649727150E-15 ) ) ;
#8798=CYLINDRICAL_SURFACE ( 'NONE', #21802, 15.00000000000000000 ) ;
#8808=CARTESIAN_POINT ( 'NONE',  ( 7.236395654485760609, 7.524999997268827734, -22.27133577429736633 ) ) ;
#8824=CARTESIAN_POINT ( 'NONE',  ( 23.41746825000000243, 13.02499999726881619, 7.608796670333735079 ) ) ;
#8850=CARTESIAN_POINT ( 'NONE',  ( -24.50000000000000711, 11.09999999999999787, 7.960532557706201828 ) ) ;
#8890=CARTESIAN_POINT ( 'NONE',  ( 24.50000000000000355, 10.10000000000000142, -7.960532557706203605 ) ) ;
#8895=CARTESIAN_POINT ( 'NONE',  ( -4.523095164977117273E-15, 8.124999997268826490, 24.62258325217400312 ) ) ;
#8896=CARTESIAN_POINT ( 'NONE',  ( 3.880418787951139592, 3.301254276084478523, 24.50000000000000000 ) ) ;
#8900=CARTESIAN_POINT ( 'NONE',  ( 19.82091636218621389, 1.949999994537626735, -14.40073868116559197 ) ) ;
#8931=CARTESIAN_POINT ( 'NONE',  ( -23.41746824999999887, 13.62499999726882116, -2.867812753649727150E-15 ) ) ;
#8941=ORIENTED_EDGE ( 'NONE', *, *, #33353, .F. ) ;
#8963=( BOUNDED_CURVE ( )  B_SPLINE_CURVE ( 2, ( #17878, #22211, #2071, #9973, #32488, #3842, #31070, #30724, #28331, #27991, #7566, #17703, #28162 ),
 .UNSPECIFIED., .F., .T. ) 
 B_SPLINE_CURVE_WITH_KNOTS ( ( 3, 2, 2, 2, 2, 2, 3 ),
 ( 0.3055555555555555802, 0.3111111111111111160, 0.3222222222222222432, 0.3333333333333333148, 0.3444444444444444420, 0.3555555555555555691, 0.3611111111111111049 ),
 .UNSPECIFIED. ) 
 CURVE ( )  GEOMETRIC_REPRESENTATION_ITEM ( )  RATIONAL_B_SPLINE_CURVE ( ( 0.9755282581475767101, 0.9755282581475768211, 1.000000000000000000, 0.9510565162951535312, 1.000000000000000000, 0.9510565162951535312, 1.000000000000000000, 0.9510565162951535312, 1.000000000000000000, 0.9510565162951535312, 1.000000000000000000, 0.9755282581475768211, 0.9755282581475768211 ) ) 
 REPRESENTATION_ITEM ( '' )  );
#8979=CARTESIAN_POINT ( 'NONE',  ( -7.236395654485757944, 7.724999997268805707, -22.27133577429736988 ) ) ;
#8995=CARTESIAN_POINT ( 'NONE',  ( 14.47279130897151767, 17.42499999726882365, -19.92008829642072598 ) ) ;
#9018=CARTESIAN_POINT ( 'NONE',  ( -19.82091636218621034, 8.549999994537621717, -14.40073868116559552 ) ) ;
#9061=CARTESIAN_POINT ( 'NONE',  ( -24.50000000000000355, 12.90000000000000036, -7.960532557706207157 ) ) ;
#9065=CARTESIAN_POINT ( 'NONE',  ( -18.94512977948576093, 9.824999997268824004, 13.76444248337722698 ) ) ;
#9070=CARTESIAN_POINT ( 'NONE',  ( 12.40046052489741157, 16.99999999999998579, -19.87944187943455177 ) ) ;
#9094=CARTESIAN_POINT ( 'NONE',  ( 19.82091636218621034, 11.80000000000000426, 14.40073868116559730 ) ) ;
#9099=CARTESIAN_POINT ( 'NONE',  ( 23.41746825000000243, 8.524999997268812635, 7.608796670333735079 ) ) ;
#9143=CARTESIAN_POINT ( 'NONE',  ( -23.41746825000000243, 10.02499999726882507, -7.608796670333730638 ) ) ;
#9158=CARTESIAN_POINT ( 'NONE',  ( -7.236395654485757944, 5.224999997268803043, -22.27133577429736988 ) ) ;
#9181=CARTESIAN_POINT ( 'NONE',  ( 7.570916362186207671, 7.349999994537615322, 23.30088464923126779 ) ) ;
#9188=DIRECTION ( 'NONE',  ( 0.000000000000000000, -1.000000000000000000, 0.000000000000000000 ) ) ;
#9194=CARTESIAN_POINT ( 'NONE',  ( 18.94512977948576093, 1.324999997268816454, -13.76444248337722875 ) ) ;
#9209=EDGE_CURVE ( 'NONE', #3518, #14369, #4052, .T. ) ;
#9226=CARTESIAN_POINT ( 'NONE',  ( -23.41746824999999887, 11.62499999726881938, -2.867812753649727150E-15 ) ) ;
#9238=CARTESIAN_POINT ( 'NONE',  ( -24.50000000000000000, 16.99999999999998579, -3.000384657911015469E-15 ) ) ;
#9261=CARTESIAN_POINT ( 'NONE',  ( 14.47279130897151589, 10.32499999726881335, 19.92008829642072953 ) ) ;
#9284=CARTESIAN_POINT ( 'NONE',  ( 1.507698388325705758E-15, 3.624999997268822938, -24.62258325217400312 ) ) ;
#9305=CARTESIAN_POINT ( 'NONE',  ( -14.47279130897152122, 4.424999997268826313, 19.92008829642072243 ) ) ;
#9318=CARTESIAN_POINT ( 'NONE',  ( -14.47279130897152122, 3.924999997268813434, 19.92008829642072243 ) ) ;
#9345=CARTESIAN_POINT ( 'NONE',  ( -4.732186688966233175E-15, 5.249999994537621895, 25.76082449383753925 ) ) ;
#9355=CARTESIAN_POINT ( 'NONE',  ( 24.50000000000000000, 2.000000000000001776, 0.000000000000000000 ) ) ;
#9356=( BOUNDED_CURVE ( )  B_SPLINE_CURVE ( 2, ( #22103, #19526, #21604, #32047, #24343, #29633, #6135, #975, #16620, #6481, #16953, #27412, #3901 ),
 .UNSPECIFIED., .F., .T. ) 
 B_SPLINE_CURVE_WITH_KNOTS ( ( 3, 2, 2, 2, 2, 2, 3 ),
 ( 0.7500000000000000000, 0.7555555555555555358, 0.7666666666666667185, 0.7777777777777777901, 0.7888888888888888618, 0.8000000000000000444, 0.8055555555555555802 ),
 .UNSPECIFIED. ) 
 CURVE ( )  GEOMETRIC_REPRESENTATION_ITEM ( )  RATIONAL_B_SPLINE_CURVE ( ( 0.9755282581475768211, 0.9755282581475768211, 1.000000000000000000, 0.9510565162951535312, 1.000000000000000000, 0.9510565162951535312, 1.000000000000000000, 0.9510565162951535312, 1.000000000000000000, 0.9510565162951535312, 1.000000000000000000, 0.9755282581475768211, 0.9755282581475768211 ) ) 
 REPRESENTATION_ITEM ( '' )  );
#9360=CARTESIAN_POINT ( 'NONE',  ( 23.41746825000000243, 5.024999997268808194, 7.608796670333735079 ) ) ;
#9374=CARTESIAN_POINT ( 'NONE',  ( -19.82091636218621389, 3.200000000000008171, 14.40073868116558842 ) ) ;
#9397=CARTESIAN_POINT ( 'NONE',  ( -22.34336606078432652, 16.99999999999999645, -9.508438583994943016 ) ) ;
#9426=SURFACE_STYLE_FILL_AREA ( #32927 ) ;
#9429=CARTESIAN_POINT ( 'NONE',  ( 18.94512977948576093, 16.82499999726880091, -13.76444248337722875 ) ) ;
#9432=CARTESIAN_POINT ( 'NONE',  ( 0.000000000000000000, 16.99999999999998579, -24.50000000000000000 ) ) ;
#9484=CARTESIAN_POINT ( 'NONE',  ( 23.41746825000000243, 7.224999997268826135, -7.608796670333727974 ) ) ;
#9499=CARTESIAN_POINT ( 'NONE',  ( 23.41746825000000243, 0.7249999972688272454, -7.608796670333727974 ) ) ;
#9516=DIRECTION ( 'NONE',  ( 0.000000000000000000, 0.000000000000000000, -1.000000000000000000 ) ) ;
#9525=CARTESIAN_POINT ( 'NONE',  ( 1.577395562988744260E-15, 6.249999994537619230, -25.76082449383753925 ) ) ;
#9533=DIRECTION ( 'NONE',  ( 0.000000000000000000, -1.000000000000000000, 0.000000000000000000 ) ) ;
#9538=CARTESIAN_POINT ( 'NONE',  ( -23.41746825000000598, 4.224999997268803931, 7.608796670333726198 ) ) ;
#9553=CARTESIAN_POINT ( 'NONE',  ( -19.82091636218621034, 8.549999994537621717, -14.40073868116559552 ) ) ;
#9610=CARTESIAN_POINT ( 'NONE',  ( -14.47279130897152122, 15.92499999726881121, 19.92008829642072243 ) ) ;
#9620=LINE ( 'NONE', #33985, #3656 ) ;
#9634=CARTESIAN_POINT ( 'NONE',  ( -7.236395654485757944, 9.724999997268806595, -22.27133577429736988 ) ) ;
#9661=CARTESIAN_POINT ( 'NONE',  ( -23.41746824999999887, 14.12499999726882294, -2.867812753649727150E-15 ) ) ;
#9675=CARTESIAN_POINT ( 'NONE',  ( 7.236395654485755280, 18.72499999726881370, 22.27133577429736988 ) ) ;
#9685=EDGE_CURVE ( 'NONE', #21231, #11786, #21528, .T. ) ;
#9699=CARTESIAN_POINT ( 'NONE',  ( -15.14183272437242600, 15.04999999453763238, 20.84094480462497856 ) ) ;
#9712=CARTESIAN_POINT ( 'NONE',  ( -4.523095164977116484E-15, 2.624999997268825158, 24.62258325217400312 ) ) ;
#9720=ORIENTED_EDGE ( 'NONE', *, *, #24746, .F. ) ;
#9724=CARTESIAN_POINT ( 'NONE',  ( -24.50000000000000711, 8.849999994537624204, 7.960532557706201828 ) ) ;
#9744=CARTESIAN_POINT ( 'NONE',  ( -4.523095164977117273E-15, 16.12499999726880517, 24.62258325217400312 ) ) ;
#9748=CARTESIAN_POINT ( 'NONE',  ( -15.12631959005131321, 16.99999999999998579, -18.67163132193408259 ) ) ;
#9763=VECTOR ( 'NONE', #13178, 1000.000000000000000 ) ;
#9777=CARTESIAN_POINT ( 'NONE',  ( 7.570916362186213000, 14.14999999453761603, -23.30088464923126423 ) ) ;
#9783=CARTESIAN_POINT ( 'NONE',  ( -18.94512977948575738, 15.42499999726881832, -13.76444248337723231 ) ) ;
#9785=MANIFOLD_SOLID_BREP ( 'Cavity1', #15578 ) ;
#9791=EDGE_CURVE ( 'NONE', #12563, #33486, #25540, .T. ) ;
#9810=CARTESIAN_POINT ( 'NONE',  ( -7.236395654485763274, 10.52499999726880198, 22.27133577429736633 ) ) ;
#9811=ORIENTED_EDGE ( 'NONE', *, *, #4319, .T. ) ;
#9833=CARTESIAN_POINT ( 'NONE',  ( -7.236395654485763274, 16.52499999726880731, 22.27133577429736633 ) ) ;
#9834=CARTESIAN_POINT ( 'NONE',  ( -18.94512977948576093, 1.824999997268816898, 13.76444248337722698 ) ) ;
#9848=CARTESIAN_POINT ( 'NONE',  ( 14.47279130897151589, 4.324999997268801799, 19.92008829642072953 ) ) ;
#9870=CARTESIAN_POINT ( 'NONE',  ( 1.577395562988744260E-15, 14.24999999453762989, -25.76082449383753925 ) ) ;
#9886=EDGE_CURVE ( 'NONE', #26574, #33508, #11712, .T. ) ;
#9887=CARTESIAN_POINT ( 'NONE',  ( -7.236395654485757944, 1.724999997268800156, -22.27133577429736988 ) ) ;
#9893=VERTEX_POINT ( 'NONE', #32642 ) ;
#9896=ORIENTED_EDGE ( 'NONE', *, *, #23857, .T. ) ;
#9921=CARTESIAN_POINT ( 'NONE',  ( -23.41746824999999887, 15.62499999726882294, -2.867812753649727150E-15 ) ) ;
#9924=CARTESIAN_POINT ( 'NONE',  ( -24.38179134483146981, 16.99999999999998934, -1.972686091485069459 ) ) ;
#9940=CARTESIAN_POINT ( 'NONE',  ( 0.000000000000000000, 16.99999999999998579, 0.000000000000000000 ) ) ;
#9957=CARTESIAN_POINT ( 'NONE',  ( 7.236395654485760609, 17.02499999726880731, -22.27133577429736633 ) ) ;
#9964=CARTESIAN_POINT ( 'NONE',  ( 0.000000000000000000, 16.99999999999998579, 0.000000000000000000 ) ) ;
#9973=CARTESIAN_POINT ( 'NONE',  ( 15.14183272437242067, 5.699999999999993960, 20.84094480462498211 ) ) ;
#9986=CARTESIAN_POINT ( 'NONE',  ( -18.94512977948576093, 6.324999997268820451, 13.76444248337722698 ) ) ;
#9993=ORIENTED_EDGE ( 'NONE', *, *, #19722, .T. ) ;
#9994=CARTESIAN_POINT ( 'NONE',  ( 19.82091636218621389, 5.949999994537630066, -14.40073868116559197 ) ) ;
#10011=CIRCLE ( 'NONE', #2333, 15.00000000000000000 ) ;
#10014=CARTESIAN_POINT ( 'NONE',  ( -4.523095164977116484E-15, 10.62499999726880695, 24.62258325217400312 ) ) ;
#10015=CARTESIAN_POINT ( 'NONE',  ( -7.236395654485763274, 2.024999997268822405, 22.27133577429736633 ) ) ;
#10027=CARTESIAN_POINT ( 'NONE',  ( 14.47279130897151767, 6.924999997268805885, -19.92008829642072598 ) ) ;
#10029=ORIENTED_EDGE ( 'NONE', *, *, #21089, .F. ) ;
#10032=AXIS2_PLACEMENT_3D ( 'NONE', #28619, #7173, #28453 ) ;
#10049=CARTESIAN_POINT ( 'NONE',  ( -24.50000000000000000, 14.74999999453763166, -3.000384657911015469E-15 ) ) ;
#10063=CARTESIAN_POINT ( 'NONE',  ( 7.236395654485755280, 8.724999997268806595, 22.27133577429736988 ) ) ;
#10098=CARTESIAN_POINT ( 'NONE',  ( 7.236395654485755280, 14.22499999726881192, 22.27133577429736988 ) ) ;
#10116=CARTESIAN_POINT ( 'NONE',  ( 3.000384657911015469E-15, 16.99999999999998579, 24.50000000000000000 ) ) ;
#10133=CARTESIAN_POINT ( 'NONE',  ( 14.47279130897151767, 16.92499999726880944, -19.92008829642072598 ) ) ;
#10157=CARTESIAN_POINT ( 'NONE',  ( 7.236395654485755280, 8.724999997268806595, 22.27133577429736988 ) ) ;
#10185=CARTESIAN_POINT ( 'NONE',  ( -7.236395654485757944, 13.72499999726881015, -22.27133577429736988 ) ) ;
#10186=CARTESIAN_POINT ( 'NONE',  ( -7.236395654485757944, 1.224999997268799712, -22.27133577429736988 ) ) ;
#10202=CARTESIAN_POINT ( 'NONE',  ( 7.236395654485755280, 8.224999997268806595, 22.27133577429736988 ) ) ;
#10224=CARTESIAN_POINT ( 'NONE',  ( -3.880418787951136483, 14.30125427608446920, -24.50000000000000000 ) ) ;
#10226=CARTESIAN_POINT ( 'NONE',  ( 7.570916362186207671, 11.34999999453761887, 23.30088464923126779 ) ) ;
#10239=CARTESIAN_POINT ( 'NONE',  ( 23.41746824999999887, 9.124999997268817609, 0.000000000000000000 ) ) ;
#10271=AXIS2_PLACEMENT_3D ( 'NONE', #25040, #24537, #6174 ) ;
#10273=LINE ( 'NONE', #15938, #9763 ) ;
#10286=EDGE_CURVE ( 'NONE', #10883, #14665, #15501, .T. ) ;
#10305=CARTESIAN_POINT ( 'NONE',  ( 19.82091636218621034, 3.799999999999998046, 14.40073868116559730 ) ) ;
#10313=DIRECTION ( 'NONE',  ( 0.000000000000000000, -1.000000000000000000, 0.000000000000000000 ) ) ;
#10326=EDGE_CURVE ( 'NONE', #12037, #17796, #13496, .T. ) ;
#10330=CARTESIAN_POINT ( 'NONE',  ( -14.47279130897152299, 6.424999997268821872, 19.92008829642072243 ) ) ;
#10346=CARTESIAN_POINT ( 'NONE',  ( 14.47279130897151589, 2.324999997268805796, 19.92008829642072953 ) ) ;
#10354=CARTESIAN_POINT ( 'NONE',  ( 23.41746825000000243, 11.22499999726881548, -7.608796670333727974 ) ) ;
#10365=CARTESIAN_POINT ( 'NONE',  ( 14.47279130897151589, 8.324999997268818674, 19.92008829642072953 ) ) ;
#10379=CARTESIAN_POINT ( 'NONE',  ( -15.14183272437242778, 7.049999994537622605, 20.84094480462497856 ) ) ;
#10384=CARTESIAN_POINT ( 'NONE',  ( -24.50000000000000711, 15.09999999999998899, 7.960532557706201828 ) ) ;
#10389=CARTESIAN_POINT ( 'NONE',  ( 7.570916362186213000, 12.14999999453761426, -23.30088464923126423 ) ) ;
#10403=CARTESIAN_POINT ( 'NONE',  ( 7.236395654485755280, 6.724999997268804819, 22.27133577429736988 ) ) ;
#10409=ORIENTED_EDGE ( 'NONE', *, *, #11255, .T. ) ;
#10439=CARTESIAN_POINT ( 'NONE',  ( 8.998893468610761559, 16.99999999999998579, -21.61938333025141290 ) ) ;
#10443=FACE_OUTER_BOUND ( 'NONE', #430, .T. ) ;
#10469=CARTESIAN_POINT ( 'NONE',  ( 24.50000000000000355, 3.899999999999992806, 7.960532557706212486 ) ) ;
#10493=CARTESIAN_POINT ( 'NONE',  ( -4.523095164977117273E-15, 12.62499999726879807, 24.62258325217400312 ) ) ;
#10501=CARTESIAN_POINT ( 'NONE',  ( 24.50000000000000000, 5.649999994537638237, 7.960532557706212486 ) ) ;
#10503=CARTESIAN_POINT ( 'NONE',  ( 0.000000000000000000, -22.99999999999999289, 0.000000000000000000 ) ) ;
#10510=CARTESIAN_POINT ( 'NONE',  ( 23.41746825000000243, 6.524999997268818852, 7.608796670333735079 ) ) ;
#10521=CARTESIAN_POINT ( 'NONE',  ( 14.47279130897151589, 16.82499999726881512, 19.92008829642072953 ) ) ;
#10533=CARTESIAN_POINT ( 'NONE',  ( 7.236395654485760609, 9.024999997268828622, -22.27133577429736633 ) ) ;
#10558=CARTESIAN_POINT ( 'NONE',  ( -14.47279130897152122, 2.424999997268802332, 19.92008829642072243 ) ) ;
#10574=CARTESIAN_POINT ( 'NONE',  ( -18.94512977948576093, 6.324999997268820451, 13.76444248337722698 ) ) ;
#10575=ORIENTED_EDGE ( 'NONE', *, *, #12841, .F. ) ;
#10621=AXIS2_PLACEMENT_3D ( 'NONE', #6337, #31906, #16815 ) ;
#10638=CARTESIAN_POINT ( 'NONE',  ( 1.577395562988744260E-15, 8.499999999999992895, -25.76082449383753925 ) ) ;
#10640=CARTESIAN_POINT ( 'NONE',  ( -7.570916362186210335, 2.349999994537638415, -23.30088464923126779 ) ) ;
#10663=CARTESIAN_POINT ( 'NONE',  ( -7.236395654485763274, 14.52499999726880553, 22.27133577429736633 ) ) ;
#10678=CARTESIAN_POINT ( 'NONE',  ( 18.94512977948575738, 6.424999997268809437, 13.76444248337723408 ) ) ;
#10700=CARTESIAN_POINT ( 'NONE',  ( 1.507698388325705758E-15, 13.12499999726881228, -24.62258325217400312 ) ) ;
#10702=ORIENTED_EDGE ( 'NONE', *, *, #10286, .F. ) ;
#10728=CARTESIAN_POINT ( 'NONE',  ( 19.82091636218621389, 17.94999999453764161, -14.40073868116559197 ) ) ;
#10742=CARTESIAN_POINT ( 'NONE',  ( -14.47279130897152122, 10.42499999726881299, 19.92008829642072243 ) ) ;
#10746=DIRECTION ( 'NONE',  ( 0.000000000000000000, 0.000000000000000000, -1.000000000000000000 ) ) ;
#10752=FACE_OUTER_BOUND ( 'NONE', #5512, .T. ) ;
#10784=DIRECTION ( 'NONE',  ( 0.000000000000000000, -1.000000000000000000, 0.000000000000000000 ) ) ;
#10804=CARTESIAN_POINT ( 'NONE',  ( 1.555960095263670572E-15, 6.499999999999994671, -24.50000000000000000 ) ) ;
#10806=AXIS2_PLACEMENT_3D ( 'NONE', #13993, #11409, #10746 ) ;
#10809=CARTESIAN_POINT ( 'NONE',  ( -7.570916362186215665, 5.399999999999987921, 23.30088464923126423 ) ) ;
#10814=CARTESIAN_POINT ( 'NONE',  ( -14.47279130897151767, 3.324999997268803131, -19.92008829642072598 ) ) ;
#10828=AXIS2_PLACEMENT_3D ( 'NONE', #18026, #22817, #15445 ) ;
#10832=CARTESIAN_POINT ( 'NONE',  ( -14.47279130897151767, 11.82499999726882578, -19.92008829642072598 ) ) ;
#10851=CARTESIAN_POINT ( 'NONE',  ( -23.41746824999999887, 7.624999997268816720, -2.867812753649727150E-15 ) ) ;
#10860=CARTESIAN_POINT ( 'NONE',  ( 23.41746825000000243, 19.02499999726880375, 7.608796670333735079 ) ) ;
#10873=CARTESIAN_POINT ( 'NONE',  ( -7.236395654485757944, 13.22499999726881015, -22.27133577429736988 ) ) ;
#10883=VERTEX_POINT ( 'NONE', #11507 ) ;
#10884=CARTESIAN_POINT ( 'NONE',  ( -3.880418787951137816, 2.301254276084479411, -24.49999999999999645 ) ) ;
#10889=CARTESIAN_POINT ( 'NONE',  ( -24.50000000000000711, 6.849999994537629533, 7.960532557706201828 ) ) ;
#10891=( BOUNDED_CURVE ( )  B_SPLINE_CURVE ( 2, ( #7984, #2840, #26350, #7647, #23273, #15728, #31494, #5072, #31657, #17962, #13309, #13136, #5246 ),
 .UNSPECIFIED., .F., .F. ) 
 B_SPLINE_CURVE_WITH_KNOTS ( ( 3, 2, 2, 2, 2, 2, 3 ),
 ( 0.3611111111111111049, 0.3666666666666666408, 0.3777777777777777679, 0.3888888888888888951, 0.4000000000000000222, 0.4111111111111110938, 0.4166666666666666852 ),
 .UNSPECIFIED. ) 
 CURVE ( )  GEOMETRIC_REPRESENTATION_ITEM ( )  RATIONAL_B_SPLINE_CURVE ( ( 0.9755282581475768211, 0.9755282581475768211, 1.000000000000000000, 0.9510565162951535312, 1.000000000000000000, 0.9510565162951535312, 1.000000000000000000, 0.9510565162951535312, 1.000000000000000000, 0.9510565162951535312, 1.000000000000000000, 0.9755282581475765991, 0.9755282581475767101 ) ) 
 REPRESENTATION_ITEM ( '' )  );
#10894=CARTESIAN_POINT ( 'NONE',  ( -19.82091636218621034, 14.80000000000000782, -14.40073868116559552 ) ) ;
#10899=CARTESIAN_POINT ( 'NONE',  ( 24.50000000000000000, 19.74999999453763877, 0.000000000000000000 ) ) ;
#10913=CARTESIAN_POINT ( 'NONE',  ( -14.47279130897151589, 15.82499999726881335, -19.92008829642072598 ) ) ;
#10952=CARTESIAN_POINT ( 'NONE',  ( -19.82091636218621389, 10.94999999453763451, 14.40073868116558842 ) ) ;
#10965=DIRECTION ( 'NONE',  ( 0.000000000000000000, -1.000000000000000000, 0.000000000000000000 ) ) ;
#10975=CARTESIAN_POINT ( 'NONE',  ( 19.82091636218621034, 5.799999999999999822, 14.40073868116559730 ) ) ;
#10980=CARTESIAN_POINT ( 'NONE',  ( 7.236395654485755280, 2.224999997268800378, 22.27133577429736988 ) ) ;
#11002=CARTESIAN_POINT ( 'NONE',  ( 7.236395654485755280, 16.72499999726881370, 22.27133577429736988 ) ) ;
#11018=CARTESIAN_POINT ( 'NONE',  ( -4.523095164977116484E-15, 8.124999997268826490, 24.62258325217400312 ) ) ;
#11040=CARTESIAN_POINT ( 'NONE',  ( -7.236395654485757944, 15.22499999726881192, -22.27133577429736988 ) ) ;
#11043=CARTESIAN_POINT ( 'NONE',  ( 19.82091636218621034, 13.80000000000000604, 14.40073868116559730 ) ) ;
#11068=CARTESIAN_POINT ( 'NONE',  ( 7.570916362186213000, 18.14999999453761959, -23.30088464923126423 ) ) ;
#11082=CARTESIAN_POINT ( 'NONE',  ( 7.236395654485760609, 17.52499999726880731, -22.27133577429736633 ) ) ;
#11091=CARTESIAN_POINT ( 'NONE',  ( -19.82091636218621389, 1.200000000000006617, 14.40073868116558842 ) ) ;
#11103=CARTESIAN_POINT ( 'NONE',  ( 23.41746824999999887, 0.8749999972688105032, 0.000000000000000000 ) ) ;
#11107=CARTESIAN_POINT ( 'NONE',  ( -15.14183272437242778, 11.29999999999999361, 20.84094480462497856 ) ) ;
#11115=CARTESIAN_POINT ( 'NONE',  ( 6.350543635241933771, 16.99999999999999289, 23.08040691491506280 ) ) ;
#11118=CARTESIAN_POINT ( 'NONE',  ( 24.50000000000000000, 11.74999999453762989, 0.000000000000000000 ) ) ;
#11135=ADVANCED_FACE ( 'NONE', ( #17865, #14939 ), #7205, .F. ) ;
#11146=CARTESIAN_POINT ( 'NONE',  ( -15.14183272437242600, 13.29999999999998650, 20.84094480462497856 ) ) ;
#11148=CARTESIAN_POINT ( 'NONE',  ( -24.50000000000001066, 8.849999994537624204, 7.960532557706201828 ) ) ;
#11150=CARTESIAN_POINT ( 'NONE',  ( 14.47279130897151944, 10.92499999726882365, -19.92008829642072598 ) ) ;
#11151=CARTESIAN_POINT ( 'NONE',  ( -7.570916362186210335, 8.599999999999996092, -23.30088464923126779 ) ) ;
#11159=CIRCLE ( 'NONE', #4014, 26.50000000000000355 ) ;
#11169=CARTESIAN_POINT ( 'NONE',  ( 23.41746824999999887, 13.02499999726881619, 7.608796670333735079 ) ) ;
#11183=CARTESIAN_POINT ( 'NONE',  ( 18.94512977948576093, 8.824999997268822227, -13.76444248337722875 ) ) ;
#11205=CARTESIAN_POINT ( 'NONE',  ( 14.47279130897151767, 12.92499999726881832, -19.92008829642072598 ) ) ;
#11229=CARTESIAN_POINT ( 'NONE',  ( 23.41746825000000243, 3.224999997268806151, -7.608796670333727974 ) ) ;
#11245=CARTESIAN_POINT ( 'NONE',  ( -14.47279130897152122, 14.42499999726880056, 19.92008829642072243 ) ) ;
#11252=EDGE_LOOP ( 'NONE', ( #2519, #20929, #16365, #14646 ) ) ;
#11255=EDGE_CURVE ( 'NONE', #16123, #6266, #32932, .T. ) ;
#11278=CYLINDRICAL_SURFACE ( 'NONE', #18430, 24.50000000000000000 ) ;
#11307=CARTESIAN_POINT ( 'NONE',  ( 1.577395562988744260E-15, 10.49999999999998757, -25.76082449383753925 ) ) ;
#11310=CARTESIAN_POINT ( 'NONE',  ( 14.47279130897151944, 8.924999997268800556, -19.92008829642072598 ) ) ;
#11315=CARTESIAN_POINT ( 'NONE',  ( 24.50000000000000000, 1.849999994537612658, -7.960532557706203605 ) ) ;
#11344=CARTESIAN_POINT ( 'NONE',  ( -7.236395654485763274, 14.02499999726880553, 22.27133577429736633 ) ) ;
#11351=ORIENTED_EDGE ( 'NONE', *, *, #33397, .F. ) ;
#11362=CIRCLE ( 'NONE', #8615, 15.00000000000000000 ) ;
#11367=CARTESIAN_POINT ( 'NONE',  ( 18.94512977948576093, 12.82499999726882578, -13.76444248337722875 ) ) ;
#11369=EDGE_LOOP ( 'NONE', ( #14102, #12296, #19625, #9896 ) ) ;
#11390=CARTESIAN_POINT ( 'NONE',  ( -18.94512977948575738, 5.924999997268809437, -13.76444248337723231 ) ) ;
#11405=CARTESIAN_POINT ( 'NONE',  ( -18.94512977948576093, 16.32499999726880091, 13.76444248337722698 ) ) ;
#11409=DIRECTION ( 'NONE',  ( 0.000000000000000000, -1.000000000000000000, 0.000000000000000000 ) ) ;
#11414=CARTESIAN_POINT ( 'NONE',  ( -19.82091636218621034, 0.7999999999999951594, -14.40073868116559552 ) ) ;
#11415=ADVANCED_FACE ( 'NONE', ( #26425 ), #25103, .T. ) ;
#11429=CYLINDRICAL_SURFACE ( 'NONE', #3135, 24.50000000000000000 ) ;
#11444=CARTESIAN_POINT ( 'NONE',  ( -15.14183272437242067, 10.44999999453763095, -20.84094480462497856 ) ) ;
#11471=CARTESIAN_POINT ( 'NONE',  ( 19.82091636218621389, 10.20000000000001528, -14.40073868116559197 ) ) ;
#11475=CARTESIAN_POINT ( 'NONE',  ( -18.94512977948575738, 9.424999997268812990, -13.76444248337723231 ) ) ;
#11476=CARTESIAN_POINT ( 'NONE',  ( -4.223320258572819786E-15, 3.499999999999996891, 24.50000000000000000 ) ) ;
#11479=CARTESIAN_POINT ( 'NONE',  ( 21.01773679462570499, 16.99999999999998934, -10.35453523078706617 ) ) ;
#11505=CARTESIAN_POINT ( 'NONE',  ( 7.236395654485760609, 13.02499999726880375, -22.27133577429736633 ) ) ;
#11507=CARTESIAN_POINT ( 'NONE',  ( 23.41746824999999887, 0.6249999972688102812, 0.000000000000000000 ) ) ;
#11529=CARTESIAN_POINT ( 'NONE',  ( 23.41746824999999887, 3.024999997268813079, 7.608796670333735079 ) ) ;
#11531=VERTEX_POINT ( 'NONE', #26805 ) ;
#11536=CARTESIAN_POINT ( 'NONE',  ( -19.82091636218621034, 2.549999994537616388, -14.40073868116559552 ) ) ;
#11552=CARTESIAN_POINT ( 'NONE',  ( -18.94512977948576093, 8.324999997268822227, 13.76444248337722698 ) ) ;
#11567=CARTESIAN_POINT ( 'NONE',  ( 24.50000000000000000, 7.849999994537627757, -7.960532557706203605 ) ) ;
#11569=CARTESIAN_POINT ( 'NONE',  ( 18.94512977948576093, 17.32499999726880446, -13.76444248337722875 ) ) ;
#11588=ADVANCED_FACE ( 'NONE', ( #26641 ), #8607, .T. ) ;
#11594=CARTESIAN_POINT ( 'NONE',  ( -24.50000000000000000, 16.64999999453763735, -7.960532557706207157 ) ) ;
#11601=CARTESIAN_POINT ( 'NONE',  ( 16.68329339294214364, 16.99999999999999289, 16.74724684563455313 ) ) ;
#11603=CARTESIAN_POINT ( 'NONE',  ( 19.82091636218621389, 11.94999999453763628, -14.40073868116559197 ) ) ;
#11635=CARTESIAN_POINT ( 'NONE',  ( -7.570916362186215665, 11.39999999999999325, 23.30088464923126423 ) ) ;
#11639=CARTESIAN_POINT ( 'NONE',  ( -18.94512977948575738, 7.424999997268811214, -13.76444248337723231 ) ) ;
#11640=CARTESIAN_POINT ( 'NONE',  ( 15.14183272437242422, 4.049999994537630599, -20.84094480462497856 ) ) ;
#11643=CARTESIAN_POINT ( 'NONE',  ( 9.706506667267825961, 16.99999999999998934, -21.32484505899611449 ) ) ;
#11664=CARTESIAN_POINT ( 'NONE',  ( -17.29030653276320351, 16.99999999999998579, 17.35785989121602668 ) ) ;
#11670=CARTESIAN_POINT ( 'NONE',  ( 19.82091636218621389, 12.19999999999998863, -14.40073868116559197 ) ) ;
#11674=CARTESIAN_POINT ( 'NONE',  ( -23.41746825000000243, 13.52499999726880198, -7.608796670333730638 ) ) ;
#11697=CARTESIAN_POINT ( 'NONE',  ( 14.47279130897151944, 3.424999997268799667, -19.92008829642072598 ) ) ;
#11712=LINE ( 'NONE', #27505, #1961 ) ;
#11719=CARTESIAN_POINT ( 'NONE',  ( -7.236395654485763274, 8.524999997268828622, 22.27133577429736633 ) ) ;
#11736=CARTESIAN_POINT ( 'NONE',  ( 18.94512977948575738, 4.424999997268807661, 13.76444248337723408 ) ) ;
#11753=DIRECTION ( 'NONE',  ( 0.000000000000000000, -1.000000000000000000, 0.000000000000000000 ) ) ;
#11760=CARTESIAN_POINT ( 'NONE',  ( 24.50000000000000355, 9.649999994537628467, 7.960532557706212486 ) ) ;
#11773=( BOUNDED_CURVE ( )  B_SPLINE_CURVE ( 2, ( #19185, #16943, #6470, #31870, #3067, #3232, #5968, #16281, #26739, #24492, #3557, #27063, #21922 ),
 .UNSPECIFIED., .F., .T. ) 
 B_SPLINE_CURVE_WITH_KNOTS ( ( 3, 2, 2, 2, 2, 2, 3 ),
 ( 0.6944444444444444198, 0.6999999999999999556, 0.7111111111111111382, 0.7222222222222222099, 0.7333333333333332815, 0.7444444444444444642, 0.7500000000000000000 ),
 .UNSPECIFIED. ) 
 CURVE ( )  GEOMETRIC_REPRESENTATION_ITEM ( )  RATIONAL_B_SPLINE_CURVE ( ( 0.9755282581475768211, 0.9755282581475768211, 1.000000000000000000, 0.9510565162951535312, 1.000000000000000000, 0.9510565162951535312, 1.000000000000000000, 0.9510565162951535312, 1.000000000000000000, 0.9510565162951535312, 1.000000000000000000, 0.9755282581475768211, 0.9755282581475768211 ) ) 
 REPRESENTATION_ITEM ( '' )  );
#11777=CARTESIAN_POINT ( 'NONE',  ( -14.47279130897151589, 3.824999997268816454, -19.92008829642072598 ) ) ;
#11786=VERTEX_POINT ( 'NONE', #2876 ) ;
#11806=CARTESIAN_POINT ( 'NONE',  ( -19.82091636218621034, 10.80000000000000426, -14.40073868116559552 ) ) ;
#11810=AXIS2_PLACEMENT_3D ( 'NONE', #3349, #5755, #18807 ) ;
#11812=CARTESIAN_POINT ( 'NONE',  ( -23.41746825000000243, 7.724999997268811036, 7.608796670333725309 ) ) ;
#11816=CARTESIAN_POINT ( 'NONE',  ( -24.50000000000000000, 16.99999999999998579, -3.000384657911015469E-15 ) ) ;
#11843=CARTESIAN_POINT ( 'NONE',  ( 1.507698388325705758E-15, 9.124999997268822938, -24.62258325217400312 ) ) ;
#11849=DIRECTION ( 'NONE',  ( 0.000000000000000000, 0.000000000000000000, -1.000000000000000000 ) ) ;
#11869=CARTESIAN_POINT ( 'NONE',  ( 18.94512977948576093, 3.324999997268818230, -13.76444248337722875 ) ) ;
#11894=CARTESIAN_POINT ( 'NONE',  ( -18.94512977948575738, 9.924999997268812990, -13.76444248337723231 ) ) ;
#11907=CARTESIAN_POINT ( 'NONE',  ( -18.94512977948575738, 5.424999997268809437, -13.76444248337723231 ) ) ;
#11933=CARTESIAN_POINT ( 'NONE',  ( 24.50000000000000000, 5.749999994537624559, 0.000000000000000000 ) ) ;
#11946=CARTESIAN_POINT ( 'NONE',  ( -4.523095164977116484E-15, 4.624999997268820273, 24.62258325217400312 ) ) ;
#11954=ORIENTED_EDGE ( 'NONE', *, *, #618, .T. ) ;
#11957=CARTESIAN_POINT ( 'NONE',  ( -24.50000000000000000, 2.899999999999995470, -7.960532557706207157 ) ) ;
#12012=CARTESIAN_POINT ( 'NONE',  ( -23.41746825000000243, 15.52499999726882507, -7.608796670333730638 ) ) ;
#12034=CARTESIAN_POINT ( 'NONE',  ( -18.94512977948575738, 1.924999997268805885, -13.76444248337723231 ) ) ;
#12037=VERTEX_POINT ( 'NONE', #27508 ) ;
#12059=CARTESIAN_POINT ( 'NONE',  ( 7.236395654485755280, 8.724999997268806595, 22.27133577429736988 ) ) ;
#12072=CARTESIAN_POINT ( 'NONE',  ( -18.94512977948575738, 1.424999997268805441, -13.76444248337723231 ) ) ;
#12073=EDGE_CURVE ( 'NONE', #31792, #23152, #32217, .T. ) ;
#12096=CARTESIAN_POINT ( 'NONE',  ( -7.570916362186215665, 15.14999999453761603, 23.30088464923126423 ) ) ;
#12098=CARTESIAN_POINT ( 'NONE',  ( -15.14183272437242600, 9.049999994537618164, 20.84094480462497856 ) ) ;
#12111=CARTESIAN_POINT ( 'NONE',  ( 23.41746825000000243, 1.224999997268811480, -7.608796670333727974 ) ) ;
#12148=CARTESIAN_POINT ( 'NONE',  ( 23.38096321367099151, 16.99999999999997868, 1.514611460525974396 ) ) ;
#12183=CARTESIAN_POINT ( 'NONE',  ( 15.14183272437242245, 2.299999999999985612, -20.84094480462497856 ) ) ;
#12189=EDGE_LOOP ( 'NONE', ( #23336, #4365 ) ) ;
#12208=CARTESIAN_POINT ( 'NONE',  ( 1.507698388325705758E-15, 7.624999997268813168, -24.62258325217400312 ) ) ;
#12215=ORIENTED_EDGE ( 'NONE', *, *, #12601, .F. ) ;
#12225=CARTESIAN_POINT ( 'NONE',  ( 0.000000000000000000, -22.99999999999999289, 0.000000000000000000 ) ) ;
#12232=CARTESIAN_POINT ( 'NONE',  ( 7.236395654485760609, 13.52499999726880553, -22.27133577429736633 ) ) ;
#12246=CARTESIAN_POINT ( 'NONE',  ( -23.41746825000000598, 1.724999997268824581, 7.608796670333726198 ) ) ;
#12268=CARTESIAN_POINT ( 'NONE',  ( -15.14183272437242778, 15.04999999453763238, 20.84094480462497856 ) ) ;
#12271=CARTESIAN_POINT ( 'NONE',  ( 19.82091636218621389, 3.949999994537628289, -14.40073868116559197 ) ) ;
#12285=CARTESIAN_POINT ( 'NONE',  ( 23.41746824999999887, 5.124999997268814056, 0.000000000000000000 ) ) ;
#12296=ORIENTED_EDGE ( 'NONE', *, *, #6732, .F. ) ;
#12327=CARTESIAN_POINT ( 'NONE',  ( -15.14183272437242778, 5.049999994537627934, 20.84094480462497856 ) ) ;
#12353=CARTESIAN_POINT ( 'NONE',  ( 19.82091636218621389, 13.94999999453763806, -14.40073868116559197 ) ) ;
#12357=CARTESIAN_POINT ( 'NONE',  ( 14.47279130897151589, 16.32499999726882933, 19.92008829642072953 ) ) ;
#12377=VECTOR ( 'NONE', #15114, 1000.000000000000000 ) ;
#12384=CARTESIAN_POINT ( 'NONE',  ( -7.236395654485763274, 8.524999997268828622, 22.27133577429736633 ) ) ;
#12399=CARTESIAN_POINT ( 'NONE',  ( -14.47279130897151589, 1.324999997268808238, -19.92008829642072598 ) ) ;
#12409=CARTESIAN_POINT ( 'NONE',  ( 7.236395654485755280, 10.72499999726880837, 22.27133577429736988 ) ) ;
#12423=CARTESIAN_POINT ( 'NONE',  ( -23.41746825000000598, 3.724999997268819918, 7.608796670333726198 ) ) ;
#12449=CARTESIAN_POINT ( 'NONE',  ( 24.50000000000000355, 11.84999999453761710, -7.960532557706203605 ) ) ;
#12462=CARTESIAN_POINT ( 'NONE',  ( -18.94512977948576093, 2.324999997268817342, 13.76444248337722698 ) ) ;
#12480=( BOUNDED_CURVE ( )  B_SPLINE_CURVE ( 2, ( #20449, #18049, #4478, #15129, #4818, #7048, #7393, #22044, #25591, #28493, #19636, #6423, #1082 ),
 .UNSPECIFIED., .F., .T. ) 
 B_SPLINE_CURVE_WITH_KNOTS ( ( 3, 2, 2, 2, 2, 2, 3 ),
 ( 0.8611111111111111605, 0.8666666666666666963, 0.8777777777777777679, 0.8888888888888888395, 0.9000000000000000222, 0.9111111111111110938, 0.9166666666666667407 ),
 .UNSPECIFIED. ) 
 CURVE ( )  GEOMETRIC_REPRESENTATION_ITEM ( )  RATIONAL_B_SPLINE_CURVE ( ( 0.9755282581475768211, 0.9755282581475770431, 1.000000000000000000, 0.9510565162951535312, 1.000000000000000000, 0.9510565162951535312, 1.000000000000000000, 0.9510565162951535312, 1.000000000000000000, 0.9510565162951535312, 1.000000000000000000, 0.9755282581475765991, 0.9755282581475768211 ) ) 
 REPRESENTATION_ITEM ( '' )  );
#12491=CARTESIAN_POINT ( 'NONE',  ( 15.14183272437241889, 15.69999999999999929, 20.84094480462498211 ) ) ;
#12496=CARTESIAN_POINT ( 'NONE',  ( -18.94512977948575738, 15.42499999726881832, -13.76444248337723231 ) ) ;
#12497=EDGE_CURVE ( 'NONE', #23152, #28001, #2590, .T. ) ;
#12529=( LENGTH_UNIT ( ) NAMED_UNIT ( * ) SI_UNIT ( .MILLI., .METRE. ) );
#12532=CARTESIAN_POINT ( 'NONE',  ( 7.236395654485755280, 16.22499999726881370, 22.27133577429736988 ) ) ;
#12551=CARTESIAN_POINT ( 'NONE',  ( 19.82091636218621389, 7.949999994537631842, -14.40073868116559197 ) ) ;
#12557=CARTESIAN_POINT ( 'NONE',  ( -18.94512977948576093, 8.324999997268822227, 13.76444248337722698 ) ) ;
#12563=VERTEX_POINT ( 'NONE', #28997 ) ;
#12564=CARTESIAN_POINT ( 'NONE',  ( 0.000000000000000000, 16.99999999999998579, 0.000000000000000000 ) ) ;
#12580=CARTESIAN_POINT ( 'NONE',  ( 18.94512977948576093, 13.32499999726879913, -13.76444248337722875 ) ) ;
#12581=CARTESIAN_POINT ( 'NONE',  ( 23.41746824999999887, 4.724999997268818142, -7.608796670333727974 ) ) ;
#12593=CARTESIAN_POINT ( 'NONE',  ( -18.94512977948576093, 7.824999997268822227, 13.76444248337722698 ) ) ;
#12601=EDGE_CURVE ( 'NONE', #19251, #5367, #7669, .T. ) ;
#12618=CARTESIAN_POINT ( 'NONE',  ( 7.570916362186213000, 16.14999999453761603, -23.30088464923126423 ) ) ;
#12631=CARTESIAN_POINT ( 'NONE',  ( 23.41746825000000243, 11.02499999726882152, 7.608796670333735079 ) ) ;
#12640=CARTESIAN_POINT ( 'NONE',  ( 15.14183272437242067, 9.699999999999985079, 20.84094480462498211 ) ) ;
#12642=CARTESIAN_POINT ( 'NONE',  ( -15.14183272437242067, 8.449999994537638059, -20.84094480462497856 ) ) ;
#12663=CARTESIAN_POINT ( 'NONE',  ( -18.94512977948576093, 15.82499999726880091, 13.76444248337722698 ) ) ;
#12685=DIRECTION ( 'NONE',  ( 0.000000000000000000, 0.000000000000000000, -1.000000000000000000 ) ) ;
#12701=CARTESIAN_POINT ( 'NONE',  ( -18.94512977948575738, 17.42499999726882010, -13.76444248337723231 ) ) ;
#12727=CARTESIAN_POINT ( 'NONE',  ( -14.47279130897152299, 8.424999997268816543, 19.92008829642072243 ) ) ;
#12736=CARTESIAN_POINT ( 'NONE',  ( 3.880418787951134707, 5.301254276084476302, 24.50000000000000000 ) ) ;
#12755=CARTESIAN_POINT ( 'NONE',  ( 18.94512977948576093, 11.32499999726882578, -13.76444248337722875 ) ) ;
#12756=CARTESIAN_POINT ( 'NONE',  ( -4.523095164977117273E-15, 6.124999997268802510, 24.62258325217400312 ) ) ;
#12768=CARTESIAN_POINT ( 'NONE',  ( -18.94512977948575738, 11.42499999726881477, -13.76444248337723231 ) ) ;
#12792=CARTESIAN_POINT ( 'NONE',  ( -19.82091636218621389, 10.94999999453763451, 14.40073868116558842 ) ) ;
#12807=CARTESIAN_POINT ( 'NONE',  ( 23.41746825000000243, 9.024999997268826846, 7.608796670333735079 ) ) ;
#12819=CIRCLE ( 'NONE', #750, 24.50000000000000000 ) ;
#12841=EDGE_CURVE ( 'NONE', #19251, #19356, #19881, .T. ) ;
#12857=ORIENTED_EDGE ( 'NONE', *, *, #27597, .F. ) ;
#12873=CARTESIAN_POINT ( 'NONE',  ( -15.14183272437241889, 6.699999999999991296, -20.84094480462497856 ) ) ;
#12885=DIRECTION ( 'NONE',  ( 0.000000000000000000, 0.000000000000000000, -1.000000000000000000 ) ) ;
#12891=CARTESIAN_POINT ( 'NONE',  ( 0.000000000000000000, 16.99999999999998579, 0.000000000000000000 ) ) ;
#12897=CARTESIAN_POINT ( 'NONE',  ( -23.41746824999999887, 8.124999997268817609, -2.867812753649727150E-15 ) ) ;
#12922=CARTESIAN_POINT ( 'NONE',  ( 14.47279130897151589, 12.82499999726882400, 19.92008829642072953 ) ) ;
#12923=CARTESIAN_POINT ( 'NONE',  ( -7.236395654485763274, 6.024999997268825958, 22.27133577429736633 ) ) ;
#12935=CARTESIAN_POINT ( 'NONE',  ( 1.507698388325705758E-15, 7.124999997268828267, -24.62258325217400312 ) ) ;
#12939=ORIENTED_EDGE ( 'NONE', *, *, #33702, .F. ) ;
#12963=CARTESIAN_POINT ( 'NONE',  ( -7.570916362186210335, 14.34999999453762065, -23.30088464923126779 ) ) ;
#12977=CARTESIAN_POINT ( 'NONE',  ( 7.236395654485760609, 5.524999997268825958, -22.27133577429736633 ) ) ;
#12990=CARTESIAN_POINT ( 'NONE',  ( -7.579748464070165821E-14, 10.49999999999999112, -24.50000000000000000 ) ) ;
#12997=CARTESIAN_POINT ( 'NONE',  ( -15.14183272437242778, 5.300000000000006040, 20.84094480462497856 ) ) ;
#13015=CARTESIAN_POINT ( 'NONE',  ( -0.5356671165000767010, 16.99999999999998224, -23.72333643937275482 ) ) ;
#13030=ORIENTED_EDGE ( 'NONE', *, *, #24060, .T. ) ;
#13045=CARTESIAN_POINT ( 'NONE',  ( -24.50000000000001066, 5.100000000000012967, 7.960532557706201828 ) ) ;
#13047=CARTESIAN_POINT ( 'NONE',  ( 15.14183272437242245, 2.049999994537635484, -20.84094480462497856 ) ) ;
#13066=CARTESIAN_POINT ( 'NONE',  ( -7.236395654485757944, 13.72499999726881015, -22.27133577429736988 ) ) ;
#13074=EDGE_CURVE ( 'NONE', #13367, #14415, #14948, .T. ) ;
#13078=PLANE ( 'NONE',  #22531 ) ;
#13084=CARTESIAN_POINT ( 'NONE',  ( 23.41746824999999887, 4.624999997268814056, 0.000000000000000000 ) ) ;
#13095=( BOUNDED_CURVE ( )  B_SPLINE_CURVE ( 2, ( #4577, #4918, #25520, #12640, #23289, #33402, #33757, #7832, #30824, #18321, #7317, #2521, #12990 ),
 .UNSPECIFIED., .F., .T. ) 
 B_SPLINE_CURVE_WITH_KNOTS ( ( 3, 2, 2, 2, 2, 2, 3 ),
 ( 0.5277777777777777901, 0.5333333333333333259, 0.5444444444444443976, 0.5555555555555555802, 0.5666666666666666519, 0.5777777777777777235, 0.5833333333333333703 ),
 .UNSPECIFIED. ) 
 CURVE ( )  GEOMETRIC_REPRESENTATION_ITEM ( )  RATIONAL_B_SPLINE_CURVE ( ( 0.9755282581475768211, 0.9755282581475768211, 1.000000000000000000, 0.9510565162951535312, 1.000000000000000000, 0.9510565162951535312, 1.000000000000000000, 0.9510565162951535312, 1.000000000000000000, 0.9510565162951535312, 1.000000000000000000, 0.9755282581475765991, 0.9755282581475768211 ) ) 
 REPRESENTATION_ITEM ( '' )  );
#13106=CARTESIAN_POINT ( 'NONE',  ( 7.236395654485755280, 6.224999997268803931, 22.27133577429736988 ) ) ;
#13113=ORIENTED_EDGE ( 'NONE', *, *, #27597, .T. ) ;
#13129=CARTESIAN_POINT ( 'NONE',  ( -15.14183272437241889, 12.44999999453762918, -20.84094480462497856 ) ) ;
#13136=CARTESIAN_POINT ( 'NONE',  ( -3.880418787951124493, 7.448745718453147369, 24.50000000000000355 ) ) ;
#13144=CARTESIAN_POINT ( 'NONE',  ( 14.47279130897151767, 7.424999997268820096, -19.92008829642072598 ) ) ;
#13178=DIRECTION ( 'NONE',  ( -0.000000000000000000, -1.000000000000000000, -0.000000000000000000 ) ) ;
#13179=DIRECTION ( 'NONE',  ( 0.000000000000000000, -1.000000000000000000, 0.000000000000000000 ) ) ;
#13207=CARTESIAN_POINT ( 'NONE',  ( 24.50000000000000355, 8.100000000000006750, -7.960532557706203605 ) ) ;
#13209=CARTESIAN_POINT ( 'NONE',  ( 19.82091636218621389, 1.949999994537626735, -14.40073868116559197 ) ) ;
#13231=VECTOR ( 'NONE', #28687, 1000.000000000000000 ) ;
#13233=CARTESIAN_POINT ( 'NONE',  ( -18.94512977948576093, 12.32499999726879913, 13.76444248337722698 ) ) ;
#13234=ORIENTED_EDGE ( 'NONE', *, *, #17536, .F. ) ;
#13251=CARTESIAN_POINT ( 'NONE',  ( 7.236395654485760609, 3.024999997268823293, -22.27133577429736633 ) ) ;
#13273=CARTESIAN_POINT ( 'NONE',  ( -23.41746825000000598, 11.72499999726880127, 7.608796670333726198 ) ) ;
#13274=DIRECTION ( 'NONE',  ( 0.000000000000000000, -1.000000000000000000, 0.000000000000000000 ) ) ;
#13283=ORIENTED_EDGE ( 'NONE', *, *, #16553, .T. ) ;
#13289=CARTESIAN_POINT ( 'NONE',  ( 3.445340210940985210E-14, 7.249999994537621895, 24.50000000000000000 ) ) ;
#13301=CARTESIAN_POINT ( 'NONE',  ( 7.570916362186207671, 19.34999999453762598, 23.30088464923126779 ) ) ;
#13309=CARTESIAN_POINT ( 'NONE',  ( -7.570916362186215665, 7.399999999999989697, 23.30088464923126423 ) ) ;
#13318=CARTESIAN_POINT ( 'NONE',  ( 1.507698388325705758E-15, 9.624999997268808727, -24.62258325217400312 ) ) ;
#13354=CARTESIAN_POINT ( 'NONE',  ( 8.094135239392500125, 17.00000000000001421, -22.02093934509174389 ) ) ;
#13367=VERTEX_POINT ( 'NONE', #28832 ) ;
#13384=CARTESIAN_POINT ( 'NONE',  ( -19.82091636218621389, 7.200000000000011724, 14.40073868116558842 ) ) ;
#13386=CARTESIAN_POINT ( 'NONE',  ( -4.732186688966233175E-15, 3.249999994537627224, 25.76082449383753925 ) ) ;
#13393=( BOUNDED_CURVE ( )  B_SPLINE_CURVE ( 2, ( #32192, #5783, #21905, #32356, #16264, #26720, #24148, #8850, #619, #11107, #21577, #32023, #26882 ),
 .UNSPECIFIED., .F., .T. ) 
 B_SPLINE_CURVE_WITH_KNOTS ( ( 3, 2, 2, 2, 2, 2, 3 ),
 ( 0.5833333333333333703, 0.5888888888888889062, 0.5999999999999999778, 0.6111111111111111605, 0.6222222222222222321, 0.6333333333333333037, 0.6388888888888889506 ),
 .UNSPECIFIED. ) 
 CURVE ( )  GEOMETRIC_REPRESENTATION_ITEM ( )  RATIONAL_B_SPLINE_CURVE ( ( 0.9755282581475768211, 0.9755282581475770431, 1.000000000000000000, 0.9510565162951535312, 1.000000000000000000, 0.9510565162951535312, 1.000000000000000000, 0.9510565162951535312, 1.000000000000000000, 0.9510565162951535312, 1.000000000000000000, 0.9755282581475765991, 0.9755282581475768211 ) ) 
 REPRESENTATION_ITEM ( '' )  );
#13394=CARTESIAN_POINT ( 'NONE',  ( 7.570916362186207671, 9.349999994537617098, 23.30088464923126779 ) ) ;
#13410=CARTESIAN_POINT ( 'NONE',  ( 14.47279130897151767, 14.82499999726881690, 19.92008829642072953 ) ) ;
#13418=ADVANCED_FACE ( 'NONE', ( #161 ), #2417, .F. ) ;
#13426=CARTESIAN_POINT ( 'NONE',  ( -14.47279130897152122, 1.924999997268818541, 19.92008829642072243 ) ) ;
#13436=CARTESIAN_POINT ( 'NONE',  ( -23.41746824999999887, 18.12499999726882649, -2.867812753649727150E-15 ) ) ;
#13449=CARTESIAN_POINT ( 'NONE',  ( -4.523095164977116484E-15, 18.12499999726882649, 24.62258325217400312 ) ) ;
#13479=CARTESIAN_POINT ( 'NONE',  ( 18.94512977948576093, 1.324999997268816454, -13.76444248337722875 ) ) ;
#13492=CARTESIAN_POINT ( 'NONE',  ( -18.94512977948576093, 14.32499999726880091, 13.76444248337722698 ) ) ;
#13496=CIRCLE ( 'NONE', #21170, 15.00000000000000000 ) ;
#13502=CARTESIAN_POINT ( 'NONE',  ( -24.50000000000000711, 1.099999999999994316, 7.960532557706201828 ) ) ;
#13537=CARTESIAN_POINT ( 'NONE',  ( 0.000000000000000000, -20.99999999999998934, 0.000000000000000000 ) ) ;
#13555=( NAMED_UNIT ( * ) SI_UNIT ( $, .STERADIAN. ) SOLID_ANGLE_UNIT ( ) );
#13560=CARTESIAN_POINT ( 'NONE',  ( -7.570916362186215665, 3.399999999999986144, 23.30088464923126423 ) ) ;
#13565=CARTESIAN_POINT ( 'NONE',  ( -7.236395654485757944, 5.224999997268803043, -22.27133577429736988 ) ) ;
#13569=CARTESIAN_POINT ( 'NONE',  ( 21.34420727114686400, 16.99999999999998934, -9.663798758747949691 ) ) ;
#13584=CARTESIAN_POINT ( 'NONE',  ( -7.236395654485757944, 15.72499999726881192, -22.27133577429736988 ) ) ;
#13599=CARTESIAN_POINT ( 'NONE',  ( -14.47279130897151589, 5.324999997268826668, -19.92008829642072598 ) ) ;
#13608=CARTESIAN_POINT ( 'NONE',  ( 23.41746825000000243, 17.02499999726880731, 7.608796670333735079 ) ) ;
#13621=CARTESIAN_POINT ( 'NONE',  ( -14.47279130897152122, 13.92499999726881654, 19.92008829642072243 ) ) ;
#13626=ADVANCED_BREP_SHAPE_REPRESENTATION ( '', ( #9785, #1376 ), #33173 ) ;
#13646=CARTESIAN_POINT ( 'NONE',  ( 15.14183272437241889, 17.44999999453761319, 20.84094480462498211 ) ) ;
#13658=CARTESIAN_POINT ( 'NONE',  ( 3.880418787951153803, 7.301254276084462091, 24.49999999999999645 ) ) ;
#13661=CARTESIAN_POINT ( 'NONE',  ( -23.41746825000000243, 18.02499999726880731, -7.608796670333730638 ) ) ;
#13664=CYLINDRICAL_SURFACE ( 'NONE', #10806, 24.50000000000000000 ) ;
#13691=CARTESIAN_POINT ( 'NONE',  ( -4.779127830720365289, 16.99999999999998224, 23.70577217035268092 ) ) ;
#13721=CARTESIAN_POINT ( 'NONE',  ( 15.14183272437242245, 12.29999999999999183, -20.84094480462497856 ) ) ;
#13723=CARTESIAN_POINT ( 'NONE',  ( -15.14183272437242600, 5.049999994537627934, 20.84094480462497856 ) ) ;
#13725=CARTESIAN_POINT ( 'NONE',  ( 1.507698388325705758E-15, 7.124999997268828267, -24.62258325217400312 ) ) ;
#13726=CARTESIAN_POINT ( 'NONE',  ( 7.570916362186207671, 3.349999994537639303, 23.30088464923126779 ) ) ;
#13729=CARTESIAN_POINT ( 'NONE',  ( 8.998893468610761559, 16.99999999999998579, -21.61938333025141290 ) ) ;
#13741=CARTESIAN_POINT ( 'NONE',  ( 21.64573397815488676, 16.99999999999998579, 8.935324268693841887 ) ) ;
#13756=CARTESIAN_POINT ( 'NONE',  ( 14.47279130897151767, 12.92499999726881832, -19.92008829642072598 ) ) ;
#13780=CARTESIAN_POINT ( 'NONE',  ( 14.47279130897151589, 18.32499999726882578, 19.92008829642072953 ) ) ;
#13808=CARTESIAN_POINT ( 'NONE',  ( -4.732186688966233175E-15, 17.24999999453762101, 25.76082449383753925 ) ) ;
#13822=DIRECTION ( 'NONE',  ( 0.000000000000000000, 0.000000000000000000, -1.000000000000000000 ) ) ;
#13824=CARTESIAN_POINT ( 'NONE',  ( 23.41746825000000243, 13.22499999726881192, -7.608796670333727974 ) ) ;
#13856=CARTESIAN_POINT ( 'NONE',  ( -9.065058954415986747, 16.99999999999998579, 22.60608526228350357 ) ) ;
#13859=CARTESIAN_POINT ( 'NONE',  ( 24.50000000000000000, 11.84999999453761710, -7.960532557706203605 ) ) ;
#13889=CARTESIAN_POINT ( 'NONE',  ( 15.14183272437241889, 11.70000000000000995, 20.84094480462498211 ) ) ;
#13892=CARTESIAN_POINT ( 'NONE',  ( -23.41746824999999887, 13.62499999726882116, -2.867812753649727150E-15 ) ) ;
#13893=CARTESIAN_POINT ( 'NONE',  ( -24.50000000000000000, 16.99999999999998579, -3.000384657911015469E-15 ) ) ;
#13897=CARTESIAN_POINT ( 'NONE',  ( 7.570916362186213000, 2.149999994537632464, -23.30088464923126423 ) ) ;
#13906=CARTESIAN_POINT ( 'NONE',  ( -7.570916362186210335, 16.60000000000000497, -23.30088464923126779 ) ) ;
#13925=CARTESIAN_POINT ( 'NONE',  ( -14.47279130897152122, 13.92499999726881654, 19.92008829642072243 ) ) ;
#13946=CARTESIAN_POINT ( 'NONE',  ( 7.236395654485755280, 14.22499999726881192, 22.27133577429736988 ) ) ;
#13950=CARTESIAN_POINT ( 'NONE',  ( -4.223320258572819786E-15, 5.249999994537629888, 24.50000000000000000 ) ) ;
#13971=CARTESIAN_POINT ( 'NONE',  ( -24.50000000000000355, 16.64999999453763735, -7.960532557706207157 ) ) ;
#13988=CARTESIAN_POINT ( 'NONE',  ( -14.47279130897151589, 13.82499999726882045, -19.92008829642072598 ) ) ;
#13992=( BOUNDED_CURVE ( )  B_SPLINE_CURVE ( 2, ( #4946, #2891, #7860, #26231, #18350, #28622, #15604, #23321, #31539, #15254, #7693, #7347, #28289 ),
 .UNSPECIFIED., .F., .T. ) 
 B_SPLINE_CURVE_WITH_KNOTS ( ( 3, 2, 2, 2, 2, 2, 3 ),
 ( 0.5833333333333333703, 0.5888888888888889062, 0.5999999999999999778, 0.6111111111111111605, 0.6222222222222222321, 0.6333333333333333037, 0.6388888888888889506 ),
 .UNSPECIFIED. ) 
 CURVE ( )  GEOMETRIC_REPRESENTATION_ITEM ( )  RATIONAL_B_SPLINE_CURVE ( ( 0.9755282581475768211, 0.9755282581475770431, 1.000000000000000000, 0.9510565162951535312, 1.000000000000000000, 0.9510565162951535312, 1.000000000000000000, 0.9510565162951535312, 1.000000000000000000, 0.9510565162951535312, 1.000000000000000000, 0.9755282581475765991, 0.9755282581475768211 ) ) 
 REPRESENTATION_ITEM ( '' )  );
#13993=CARTESIAN_POINT ( 'NONE',  ( 0.000000000000000000, 16.99999999999998579, 0.000000000000000000 ) ) ;
#13996=VERTEX_POINT ( 'NONE', #19554 ) ;
#14012=FACE_OUTER_BOUND ( 'NONE', #11252, .T. ) ;
#14019=CARTESIAN_POINT ( 'NONE',  ( 5.411497909691496133, 16.99999999999998934, 23.34105529868805817 ) ) ;
#14027=CARTESIAN_POINT ( 'NONE',  ( -3.712076227271900841E-14, 10.24999999453763344, -24.50000000000000000 ) ) ;
#14054=CARTESIAN_POINT ( 'NONE',  ( 24.50000000000000355, 14.09999999999999254, -7.960532557706203605 ) ) ;
#14058=CARTESIAN_POINT ( 'NONE',  ( 7.236395654485755280, 8.224999997268806595, 22.27133577429736988 ) ) ;
#14059=CARTESIAN_POINT ( 'NONE',  ( -3.880418787951156023, 8.551254281546841085, -24.49999999999999645 ) ) ;
#14095=CARTESIAN_POINT ( 'NONE',  ( 23.41746824999999887, 8.624999997268817609, 0.000000000000000000 ) ) ;
#14102=ORIENTED_EDGE ( 'NONE', *, *, #16824, .T. ) ;
#14115=CARTESIAN_POINT ( 'NONE',  ( -23.41746824999999887, 17.62499999726882649, -2.867812753649727150E-15 ) ) ;
#14127=ORIENTED_EDGE ( 'NONE', *, *, #19722, .F. ) ;
#14142=CARTESIAN_POINT ( 'NONE',  ( -4.523095164977116484E-15, 4.624999997268820273, 24.62258325217400312 ) ) ;
#14156=CARTESIAN_POINT ( 'NONE',  ( -7.236395654485757944, 15.72499999726881192, -22.27133577429736988 ) ) ;
#14179=CARTESIAN_POINT ( 'NONE',  ( -17.29030653276319995, 16.99999999999998579, 17.35785989121602668 ) ) ;
#14205=VERTEX_POINT ( 'NONE', #33950 ) ;
#14223=CARTESIAN_POINT ( 'NONE',  ( -24.50000000000000355, 10.90000000000000568, -7.960532557706207157 ) ) ;
#14227=CARTESIAN_POINT ( 'NONE',  ( -7.236395654485757944, 11.22499999726880837, -22.27133577429736988 ) ) ;
#14228=CARTESIAN_POINT ( 'NONE',  ( 24.50000000000000000, 3.849999994537637082, -7.960532557706203605 ) ) ;
#14245=EDGE_LOOP ( 'NONE', ( #33003, #28629, #1263, #16525, #19460, #30393, #4000, #9720 ) ) ;
#14254=CARTESIAN_POINT ( 'NONE',  ( 24.50000000000000000, 12.09999999999999609, -7.960532557706203605 ) ) ;
#14258=CARTESIAN_POINT ( 'NONE',  ( 23.41746824999999887, 14.62499999726882294, 0.000000000000000000 ) ) ;
#14267=ORIENTED_EDGE ( 'NONE', *, *, #9791, .T. ) ;
#14285=CARTESIAN_POINT ( 'NONE',  ( 7.236395654485755280, 4.724999997268803043, 22.27133577429736988 ) ) ;
#14290=ORIENTED_EDGE ( 'NONE', *, *, #4893, .T. ) ;
#14307=CARTESIAN_POINT ( 'NONE',  ( -23.41746825000000243, 6.024999997268805529, -7.608796670333730638 ) ) ;
#14322=CARTESIAN_POINT ( 'NONE',  ( -18.94512977948576093, 1.824999997268816898, 13.76444248337722698 ) ) ;
#14328=ORIENTED_EDGE ( 'NONE', *, *, #32304, .T. ) ;
#14347=CARTESIAN_POINT ( 'NONE',  ( -4.732186688966233175E-15, 9.249999994537640546, 25.76082449383753925 ) ) ;
#14353=CARTESIAN_POINT ( 'NONE',  ( -17.29030653276320351, 16.99999999999998579, 17.35785989121602668 ) ) ;
#14360=CARTESIAN_POINT ( 'NONE',  ( -19.82091636218621034, 10.54999999453762349, -14.40073868116559552 ) ) ;
#14366=ORIENTED_EDGE ( 'NONE', *, *, #15463, .F. ) ;
#14369=VERTEX_POINT ( 'NONE', #31028 ) ;
#14388=CARTESIAN_POINT ( 'NONE',  ( 7.570916362186207671, 11.59999999999999964, 23.30088464923126779 ) ) ;
#14393=CARTESIAN_POINT ( 'NONE',  ( 18.94512977948576093, 8.824999997268822227, -13.76444248337722875 ) ) ;
#14398=CARTESIAN_POINT ( 'NONE',  ( -8.705037036007741591, 16.99999999999998224, -22.19839023265693356 ) ) ;
#14415=VERTEX_POINT ( 'NONE', #23320 ) ;
#14428=CARTESIAN_POINT ( 'NONE',  ( 23.41746825000000243, 8.724999997268806595, -7.608796670333727974 ) ) ;
#14474=CARTESIAN_POINT ( 'NONE',  ( 7.236395654485760609, 5.524999997268825958, -22.27133577429736633 ) ) ;
#14489=CARTESIAN_POINT ( 'NONE',  ( 23.41746824999999887, 19.12499999726882649, 0.000000000000000000 ) ) ;
#14513=CARTESIAN_POINT ( 'NONE',  ( 24.50000000000000355, 3.649999994537613812, 7.960532557706212486 ) ) ;
#14522=( BOUNDED_CURVE ( )  B_SPLINE_CURVE ( 2, ( #4697, #17932, #7447, #4871, #11043, #8452, #26655, #31461, #20844, #18942, #21509, #29387, #18610 ),
 .UNSPECIFIED., .F., .T. ) 
 B_SPLINE_CURVE_WITH_KNOTS ( ( 3, 2, 2, 2, 2, 2, 3 ),
 ( 0.7500000000000000000, 0.7555555555555555358, 0.7666666666666667185, 0.7777777777777777901, 0.7888888888888888618, 0.8000000000000000444, 0.8055555555555555802 ),
 .UNSPECIFIED. ) 
 CURVE ( )  GEOMETRIC_REPRESENTATION_ITEM ( )  RATIONAL_B_SPLINE_CURVE ( ( 0.9755282581475768211, 0.9755282581475768211, 1.000000000000000000, 0.9510565162951535312, 1.000000000000000000, 0.9510565162951535312, 1.000000000000000000, 0.9510565162951535312, 1.000000000000000000, 0.9510565162951535312, 1.000000000000000000, 0.9755282581475768211, 0.9755282581475768211 ) ) 
 REPRESENTATION_ITEM ( '' )  );
#14556=CARTESIAN_POINT ( 'NONE',  ( -24.50000000000000355, 16.89999999999998437, -7.960532557706207157 ) ) ;
#14562=CARTESIAN_POINT ( 'NONE',  ( 14.47279130897151767, 8.324999997268818674, 19.92008829642072953 ) ) ;
#14566=CARTESIAN_POINT ( 'NONE',  ( -10.52618891537850310, 16.99999999999997868, -21.44545275267361006 ) ) ;
#14580=EDGE_LOOP ( 'NONE', ( #2339, #26238, #2727, #28172 ) ) ;
#14598=CARTESIAN_POINT ( 'NONE',  ( 24.50000000000000000, 2.000000000000001776, 0.000000000000000000 ) ) ;
#14621=CARTESIAN_POINT ( 'NONE',  ( -7.236395654485763274, 2.524999997268823293, 22.27133577429736633 ) ) ;
#14624=ORIENTED_EDGE ( 'NONE', *, *, #9791, .F. ) ;
#14627=ORIENTED_EDGE ( 'NONE', *, *, #5280, .F. ) ;
#14641=CARTESIAN_POINT ( 'NONE',  ( 3.880418787951153803, 7.551254281546842861, 24.49999999999999645 ) ) ;
#14644=B_SPLINE_CURVE_WITH_KNOTS ( 'NONE', 3,
 ( #11816, #4601, #33427, #9924, #25369, #30674, #32898, #17485, #17147, #20400, #9397, #22292, #27600, #22797, #33252, #19880, #30333, #9748, #7343, #20234, #19714, #14566, #17828, #3924, #14398, #6830, #21258, #13015, #23486, #21090, #26226, #294, #33947, #5289, #13354, #10439 ),
 .UNSPECIFIED., .F., .F.,
 ( 4, 2, 2, 2, 2, 2, 2, 2, 2, 2, 2, 2, 2, 2, 2, 2, 2, 4 ),
 ( 0.000000000000000000, 0.001481992817026406284, 0.002963985634052812568, 0.005927971268105625136, 0.008891956902158437703, 0.01037394971918484572, 0.01185594253621125548, 0.01778391380431686847, 0.02074789943836967063, 0.02371188507242247626, 0.02667587070647528535, 0.02815786352350169164, 0.02963985634052809445, 0.03556782760863372306, 0.04149579887673936207, 0.04297779169376576835, 0.04445978451079217464, 0.04742377014484498721 ),
 .UNSPECIFIED. ) ;
#14646=ORIENTED_EDGE ( 'NONE', *, *, #3287, .T. ) ;
#14647=CARTESIAN_POINT ( 'NONE',  ( -23.41746824999999887, 4.124999997268813168, -2.867812753649727150E-15 ) ) ;
#14659=CARTESIAN_POINT ( 'NONE',  ( -18.94512977948576093, 5.824999997268820451, 13.76444248337722698 ) ) ;
#14665=VERTEX_POINT ( 'NONE', #5210 ) ;
#14683=CARTESIAN_POINT ( 'NONE',  ( 15.14183272437241889, 7.449999994537639836, 20.84094480462498211 ) ) ;
#14694=CARTESIAN_POINT ( 'NONE',  ( -6.668400408272875007E-16, 2.249999994537632553, -24.50000000000000355 ) ) ;
#14705=ORIENTED_EDGE ( 'NONE', *, *, #549, .T. ) ;
#14711=CARTESIAN_POINT ( 'NONE',  ( -3.880418787951142701, 3.448745718453150477, 24.49999999999999645 ) ) ;
#14730=DIRECTION ( 'NONE',  ( 0.000000000000000000, -1.000000000000000000, 0.000000000000000000 ) ) ;
#14746=ORIENTED_EDGE ( 'NONE', *, *, #24795, .T. ) ;
#14755=FACE_OUTER_BOUND ( 'NONE', #30607, .T. ) ;
#14762=SURFACE_SIDE_STYLE ('',( #9426 ) ) ;
#14765=CARTESIAN_POINT ( 'NONE',  ( -14.47279130897151589, 15.32499999726880269, -19.92008829642072598 ) ) ;
#14789=CARTESIAN_POINT ( 'NONE',  ( -18.94512977948576093, 4.324999997268818674, 13.76444248337722698 ) ) ;
#14796=ORIENTED_EDGE ( 'NONE', *, *, #20914, .F. ) ;
#14811=CARTESIAN_POINT ( 'NONE',  ( 3.445340210940985210E-14, 7.499999999999994671, 24.50000000000000000 ) ) ;
#14814=CARTESIAN_POINT ( 'NONE',  ( -14.47279130897151589, 13.82499999726882045, -19.92008829642072598 ) ) ;
#14829=CARTESIAN_POINT ( 'NONE',  ( -23.41746825000000243, 1.524999997268801755, -7.608796670333730638 ) ) ;
#14840=VERTEX_POINT ( 'NONE', #32250 ) ;
#14853=CARTESIAN_POINT ( 'NONE',  ( 19.82091636218621034, 3.549999994537617276, 14.40073868116559730 ) ) ;
#14860=DIRECTION ( 'NONE',  ( 0.000000000000000000, -1.000000000000000000, 0.000000000000000000 ) ) ;
#14896=CARTESIAN_POINT ( 'NONE',  ( 19.82091636218621034, 17.80000000000001137, 14.40073868116559730 ) ) ;
#14937=CARTESIAN_POINT ( 'NONE',  ( -18.94512977948576093, 15.82499999726880091, 13.76444248337722698 ) ) ;
#14939=FACE_OUTER_BOUND ( 'NONE', #1096, .T. ) ;
#14948=CIRCLE ( 'NONE', #10032, 26.50000000000000355 ) ;
#14963=CARTESIAN_POINT ( 'NONE',  ( 18.94512977948575738, 6.924999997268810326, 13.76444248337723408 ) ) ;
#14985=CARTESIAN_POINT ( 'NONE',  ( 14.47279130897151767, 11.42499999726880944, -19.92008829642072598 ) ) ;
#14986=CARTESIAN_POINT ( 'NONE',  ( 23.41746824999999887, 0.7249999972688272454, -7.608796670333727974 ) ) ;
#15001=CARTESIAN_POINT ( 'NONE',  ( 23.41746825000000243, 2.524999997268798868, 7.608796670333735079 ) ) ;
#15029=CARTESIAN_POINT ( 'NONE',  ( -4.732186688966233175E-15, 13.24999999453763166, 25.76082449383753925 ) ) ;
#15038=CARTESIAN_POINT ( 'NONE',  ( 19.82091636218621389, 2.200000000000007283, -14.40073868116559197 ) ) ;
#15043=CARTESIAN_POINT ( 'NONE',  ( 7.236395654485760609, 1.524999997268822183, -22.27133577429736633 ) ) ;
#15045=CARTESIAN_POINT ( 'NONE',  ( 0.000000000000000000, 16.99999999999998579, 0.000000000000000000 ) ) ;
#15075=CARTESIAN_POINT ( 'NONE',  ( -7.236395654485763274, 14.02499999726880553, 22.27133577429736633 ) ) ;
#15078=CARTESIAN_POINT ( 'NONE',  ( -7.570916362186210335, 4.349999994537640191, -23.30088464923126779 ) ) ;
#15094=( BOUNDED_CURVE ( )  B_SPLINE_CURVE ( 2, ( #3188, #13658, #1427, #4012, #2075, #6588, #32825, #11567, #12551, #32661, #23022, #22047, #3845 ),
 .UNSPECIFIED., .F., .T. ) 
 B_SPLINE_CURVE_WITH_KNOTS ( ( 3, 2, 2, 2, 2, 2, 3 ),
 ( 0.3055555555555555802, 0.3111111111111111160, 0.3222222222222222432, 0.3333333333333333148, 0.3444444444444444420, 0.3555555555555555691, 0.3611111111111111049 ),
 .UNSPECIFIED. ) 
 CURVE ( )  GEOMETRIC_REPRESENTATION_ITEM ( )  RATIONAL_B_SPLINE_CURVE ( ( 0.9755282581475767101, 0.9755282581475768211, 1.000000000000000000, 0.9510565162951535312, 1.000000000000000000, 0.9510565162951535312, 1.000000000000000000, 0.9510565162951535312, 1.000000000000000000, 0.9510565162951535312, 1.000000000000000000, 0.9755282581475768211, 0.9755282581475768211 ) ) 
 REPRESENTATION_ITEM ( '' )  );
#15095=DIRECTION ( 'NONE',  ( 0.000000000000000000, -1.000000000000000000, 0.000000000000000000 ) ) ;
#15109=( NAMED_UNIT ( * ) SI_UNIT ( $, .STERADIAN. ) SOLID_ANGLE_UNIT ( ) );
#15112=CARTESIAN_POINT ( 'NONE',  ( -19.82091636218621034, 0.7999999999999951594, -14.40073868116559552 ) ) ;
#15114=DIRECTION ( 'NONE',  ( 0.000000000000000000, -1.000000000000000000, 0.000000000000000000 ) ) ;
#15129=CARTESIAN_POINT ( 'NONE',  ( 15.14183272437242067, 15.69999999999999929, 20.84094480462498211 ) ) ;
#15139=CARTESIAN_POINT ( 'NONE',  ( -14.47279130897151767, 5.824999997268811569, -19.92008829642072598 ) ) ;
#15162=CARTESIAN_POINT ( 'NONE',  ( -18.94512977948575738, 11.92499999726881477, -13.76444248337723231 ) ) ;
#15163=CARTESIAN_POINT ( 'NONE',  ( -18.94512977948576093, 3.824999997268818674, 13.76444248337722698 ) ) ;
#15176=CARTESIAN_POINT ( 'NONE',  ( 14.47279130897151589, 12.32499999726880802, 19.92008829642072953 ) ) ;
#15200=CARTESIAN_POINT ( 'NONE',  ( 1.577395562988744260E-15, 12.24999999453763522, -25.76082449383753925 ) ) ;
#15213=CARTESIAN_POINT ( 'NONE',  ( 7.236395654485760609, 9.524999997268828622, -22.27133577429736633 ) ) ;
#15241=CARTESIAN_POINT ( 'NONE',  ( 1.577395562988744260E-15, 16.50000000000000000, -25.76082449383753925 ) ) ;
#15246=DIRECTION ( 'NONE',  ( 0.000000000000000000, 0.000000000000000000, -1.000000000000000000 ) ) ;
#15254=CARTESIAN_POINT ( 'NONE',  ( -15.14183272437242778, 13.04999999453763770, 20.84094480462497856 ) ) ;
#15277=CARTESIAN_POINT ( 'NONE',  ( 1.555960095263670572E-15, 14.24999999453762278, -24.50000000000000000 ) ) ;
#15282=CARTESIAN_POINT ( 'NONE',  ( -24.50000000000001066, 1.099999999999994094, 7.960532557706201828 ) ) ;
#15308=CARTESIAN_POINT ( 'NONE',  ( -23.41746824999999887, 6.124999997268814944, -2.867812753649727150E-15 ) ) ;
#15318=CARTESIAN_POINT ( 'NONE',  ( -4.223320258572819786E-15, 15.24999999453762278, 24.50000000000000000 ) ) ;
#15336=CARTESIAN_POINT ( 'NONE',  ( -23.41746825000000243, 14.02499999726881263, -7.608796670333730638 ) ) ;
#15337=CARTESIAN_POINT ( 'NONE',  ( 7.236395654485760609, 5.024999997268825069, -22.27133577429736633 ) ) ;
#15350=CARTESIAN_POINT ( 'NONE',  ( -7.236395654485757944, 7.224999997268804819, -22.27133577429736988 ) ) ;
#15353=ORIENTED_EDGE ( 'NONE', *, *, #15453, .T. ) ;
#15372=CARTESIAN_POINT ( 'NONE',  ( -15.14183272437242067, 14.44999999453762207, -20.84094480462497856 ) ) ;
#15374=CARTESIAN_POINT ( 'NONE',  ( 7.570916362186213000, 10.14999999453763913, -23.30088464923126423 ) ) ;
#15388=CARTESIAN_POINT ( 'NONE',  ( 1.507698388325705758E-15, 5.624999997268818497, -24.62258325217400312 ) ) ;
#15406=CARTESIAN_POINT ( 'NONE',  ( -1.756012107511856980E-14, 4.499999999999997335, -24.50000000000000000 ) ) ;
#15421=CARTESIAN_POINT ( 'NONE',  ( 6.001560367445586717E-15, 1.500000000000005995, 24.50000000000000000 ) ) ;
#15428=CYLINDRICAL_SURFACE ( 'NONE', #27046, 24.50000000000000000 ) ;
#15429=CARTESIAN_POINT ( 'NONE',  ( 23.41746824999999887, 1.124999997268810725, 0.000000000000000000 ) ) ;
#15442=ORIENTED_EDGE ( 'NONE', *, *, #31693, .F. ) ;
#15445=DIRECTION ( 'NONE',  ( 0.000000000000000000, -0.000000000000000000, -1.000000000000000000 ) ) ;
#15453=EDGE_CURVE ( 'NONE', #9893, #19228, #18334, .T. ) ;
#15456=CARTESIAN_POINT ( 'NONE',  ( 24.50000000000000355, 7.900000000000012790, 7.960532557706212486 ) ) ;
#15463=EDGE_CURVE ( 'NONE', #21102, #2430, #1952, .T. ) ;
#15482=CARTESIAN_POINT ( 'NONE',  ( -4.523095164977117273E-15, 6.624999997268815832, 24.62258325217400312 ) ) ;
#15483=ORIENTED_EDGE ( 'NONE', *, *, #32495, .F. ) ;
#15498=CARTESIAN_POINT ( 'NONE',  ( 1.507698388325705758E-15, 1.124999997268814722, -24.62258325217400312 ) ) ;
#15501=LINE ( 'NONE', #33329, #5256 ) ;
#15510=CARTESIAN_POINT ( 'NONE',  ( 23.41746825000000243, 15.22499999726880482, -7.608796670333727974 ) ) ;
#15511=CARTESIAN_POINT ( 'NONE',  ( -4.523095164977117273E-15, 2.124999997268811835, 24.62258325217400312 ) ) ;
#15521=ADVANCED_FACE ( 'NONE', ( #14012 ), #11429, .T. ) ;
#15524=CARTESIAN_POINT ( 'NONE',  ( -23.41746824999999887, 9.624999997268817609, -2.867812753649727150E-15 ) ) ;
#15549=CARTESIAN_POINT ( 'NONE',  ( 19.82091636218621389, 13.94999999453763806, -14.40073868116559197 ) ) ;
#15566=CARTESIAN_POINT ( 'NONE',  ( -7.236395654485757944, 11.72499999726880837, -22.27133577429736988 ) ) ;
#15578=CLOSED_SHELL ( 'NONE', ( #32109, #6837, #23925, #5470, #24466, #5671, #27938, #30632, #17060, #30265, #33106, #31078, #3485, #7471, #1463, #15521, #11588, #28510, #2681, #328, #19539, #11135, #20714, #3564, #22864, #19843, #11415, #13418 ) ) ;
#15592=CARTESIAN_POINT ( 'NONE',  ( -3.712076227271900841E-14, 8.499999999999994671, -24.50000000000000000 ) ) ;
#15604=CARTESIAN_POINT ( 'NONE',  ( -24.50000000000000000, 12.74999999453763166, -3.000384657911015469E-15 ) ) ;
#15607=EDGE_CURVE ( 'NONE', #16123, #26574, #13393, .T. ) ;
#15633=CARTESIAN_POINT ( 'NONE',  ( -24.50000000000001066, 3.099999999999989875, 7.960532557706201828 ) ) ;
#15649=AXIS2_PLACEMENT_3D ( 'NONE', #15045, #4055, #19844 ) ;
#15657=CARTESIAN_POINT ( 'NONE',  ( 14.47279130897151767, 16.82499999726881157, 19.92008829642072953 ) ) ;
#15658=ORIENTED_EDGE ( 'NONE', *, *, #32821, .F. ) ;
#15666=CARTESIAN_POINT ( 'NONE',  ( 1.555960095263670572E-15, 8.249999994537619230, -24.50000000000000000 ) ) ;
#15668=FACE_BOUND ( 'NONE', #12189, .T. ) ;
#15676=CARTESIAN_POINT ( 'NONE',  ( -14.47279130897152122, 3.924999997268813434, 19.92008829642072243 ) ) ;
#15684=CARTESIAN_POINT ( 'NONE',  ( -23.41746825000000598, 18.22499999726882436, 7.608796670333726198 ) ) ;
#15695=CARTESIAN_POINT ( 'NONE',  ( 1.507698388325705758E-15, 11.12499999726881761, -24.62258325217400312 ) ) ;
#15716=CARTESIAN_POINT ( 'NONE',  ( -15.14183272437242067, 14.70000000000000107, -20.84094480462497856 ) ) ;
#15721=CARTESIAN_POINT ( 'NONE',  ( 1.577395562988744260E-15, 10.24999999453763877, -25.76082449383753925 ) ) ;
#15728=CARTESIAN_POINT ( 'NONE',  ( -24.50000000000000000, 6.900000000000014566, -7.960532557706207157 ) ) ;
#15735=CARTESIAN_POINT ( 'NONE',  ( -4.523095164977116484E-15, 8.624999997268810503, 24.62258325217400312 ) ) ;
#15784=ORIENTED_EDGE ( 'NONE', *, *, #1373, .T. ) ;
#15799=CARTESIAN_POINT ( 'NONE',  ( -4.732186688966233175E-15, 7.499999999999995559, 25.76082449383753925 ) ) ;
#15801=CARTESIAN_POINT ( 'NONE',  ( 24.50000000000000000, 1.749999994537621006, 0.000000000000000000 ) ) ;
#15824=CARTESIAN_POINT ( 'NONE',  ( -18.94512977948575738, 13.92499999726881654, -13.76444248337723231 ) ) ;
#15832=CYLINDRICAL_SURFACE ( 'NONE', #31915, 24.50000000000000000 ) ;
#15839=CARTESIAN_POINT ( 'NONE',  ( -7.236395654485757944, 5.224999997268803043, -22.27133577429736988 ) ) ;
#15849=CARTESIAN_POINT ( 'NONE',  ( 23.41746824999999887, 17.12499999726882649, 0.000000000000000000 ) ) ;
#15861=CARTESIAN_POINT ( 'NONE',  ( -7.236395654485757944, 9.224999997268806595, -22.27133577429736988 ) ) ;
#15879=CARTESIAN_POINT ( 'NONE',  ( 0.000000000000000000, 16.99999999999998579, -24.50000000000000000 ) ) ;
#15881=CARTESIAN_POINT ( 'NONE',  ( 1.555960095263670572E-15, 14.50000000000000178, -24.50000000000000000 ) ) ;
#15887=CARTESIAN_POINT ( 'NONE',  ( 23.41746825000000243, 1.224999997268811480, -7.608796670333727974 ) ) ;
#15902=CARTESIAN_POINT ( 'NONE',  ( 14.47279130897151589, 8.824999997268804464, 19.92008829642072953 ) ) ;
#15938=CARTESIAN_POINT ( 'NONE',  ( 1.836970198721029589E-15, 16.99999999999998579, 15.00000000000000000 ) ) ;
#15943=CARTESIAN_POINT ( 'NONE',  ( 24.50000000000000000, 1.749999994537621006, 0.000000000000000000 ) ) ;
#15952=ORIENTED_EDGE ( 'NONE', *, *, #5240, .F. ) ;
#15967=CARTESIAN_POINT ( 'NONE',  ( 24.50000000000000355, 5.899999999999987921, 7.960532557706212486 ) ) ;
#15969=CARTESIAN_POINT ( 'NONE',  ( -7.570916362186215665, 3.149999994537633352, 23.30088464923126423 ) ) ;
#15992=CARTESIAN_POINT ( 'NONE',  ( 18.94512977948575738, 16.92499999726882010, 13.76444248337723408 ) ) ;
#16003=VECTOR ( 'NONE', #31976, 1000.000000000000000 ) ;
#16009=CARTESIAN_POINT ( 'NONE',  ( -14.47279130897151589, 7.324999997268822227, -19.92008829642072598 ) ) ;
#16031=CARTESIAN_POINT ( 'NONE',  ( 23.41746825000000243, 14.52499999726882685, 7.608796670333735079 ) ) ;
#16042=AXIS2_PLACEMENT_3D ( 'NONE', #30856, #7349, #4777 ) ;
#16058=CARTESIAN_POINT ( 'NONE',  ( -7.236395654485757944, 3.724999997268802154, -22.27133577429736988 ) ) ;
#16073=CARTESIAN_POINT ( 'NONE',  ( 23.41746825000000243, 15.22499999726880482, -7.608796670333727974 ) ) ;
#16090=EDGE_CURVE ( 'NONE', #1393, #4913, #19422, .T. ) ;
#16123=VERTEX_POINT ( 'NONE', #3302 ) ;
#16138=CARTESIAN_POINT ( 'NONE',  ( 1.577395562988744260E-15, 6.499999999999998224, -25.76082449383753925 ) ) ;
#16144=CARTESIAN_POINT ( 'NONE',  ( 1.507698388325705758E-15, 5.124999997268805174, -24.62258325217400312 ) ) ;
#16145=CARTESIAN_POINT ( 'NONE',  ( 15.14183272437242067, 3.699999999999999289, 20.84094480462498211 ) ) ;
#16161=CARTESIAN_POINT ( 'NONE',  ( -14.47279130897151767, 13.82499999726882045, -19.92008829642072598 ) ) ;
#16173=CARTESIAN_POINT ( 'NONE',  ( 7.313012447739250820E-14, 13.24999999453762456, 24.50000000000000000 ) ) ;
#16177=CARTESIAN_POINT ( 'NONE',  ( 23.41746825000000243, 4.524999997268823293, 7.608796670333735079 ) ) ;
#16200=CARTESIAN_POINT ( 'NONE',  ( 23.41746824999999887, 12.62499999726882116, 0.000000000000000000 ) ) ;
#16227=CARTESIAN_POINT ( 'NONE',  ( 24.50000000000000355, 19.64999999453763024, 7.960532557706212486 ) ) ;
#16239=CARTESIAN_POINT ( 'NONE',  ( -14.47279130897152122, 16.42499999726882365, 19.92008829642072243 ) ) ;
#16263=PRODUCT_DEFINITION ( 'UNKNOWN', '', #6596, #29493 ) ;
#16264=CARTESIAN_POINT ( 'NONE',  ( -19.82091636218621034, 10.80000000000000426, -14.40073868116559552 ) ) ;
#16271=CARTESIAN_POINT ( 'NONE',  ( 13.39151655733673607, 16.99999999999997158, 19.69815938956502066 ) ) ;
#16281=CARTESIAN_POINT ( 'NONE',  ( -24.50000000000000711, 13.09999999999999432, 7.960532557706201828 ) ) ;
#16302=CARTESIAN_POINT ( 'NONE',  ( -4.732186688966233175E-15, 9.499999999999991118, 25.76082449383753925 ) ) ;
#16305=CARTESIAN_POINT ( 'NONE',  ( 1.577395562988744260E-15, 8.249999994537613901, -25.76082449383753925 ) ) ;
#16308=CARTESIAN_POINT ( 'NONE',  ( 14.47279130897151944, 6.924999997268805885, -19.92008829642072598 ) ) ;
#16326=CARTESIAN_POINT ( 'NONE',  ( -23.41746824999999887, 16.02499999726881086, -7.608796670333730638 ) ) ;
#16327=ORIENTED_EDGE ( 'NONE', *, *, #12841, .T. ) ;
#16341=CARTESIAN_POINT ( 'NONE',  ( 14.47279130897151767, 6.924999997268805885, -19.92008829642072598 ) ) ;
#16363=CARTESIAN_POINT ( 'NONE',  ( -23.41746825000000243, 17.52499999726881796, -7.608796670333730638 ) ) ;
#16365=ORIENTED_EDGE ( 'NONE', *, *, #9685, .T. ) ;
#16389=CARTESIAN_POINT ( 'NONE',  ( 7.570916362186207671, 17.34999999453762243, 23.30088464923126779 ) ) ;
#16404=CARTESIAN_POINT ( 'NONE',  ( -18.94512977948576093, 12.32499999726879913, 13.76444248337722698 ) ) ;
#16408=( BOUNDED_CURVE ( )  B_SPLINE_CURVE ( 2, ( #26935, #3433, #13906, #24372, #844, #29664, #9238 ),
 .UNSPECIFIED., .F., .T. ) 
 B_SPLINE_CURVE_WITH_KNOTS ( ( 3, 2, 2, 3 ),
 ( 0.9166666666666667407, 0.9222222222222221655, 0.9333333333333329040, 0.9444444444444436426 ),
 .UNSPECIFIED. ) 
 CURVE ( )  GEOMETRIC_REPRESENTATION_ITEM ( )  RATIONAL_B_SPLINE_CURVE ( ( 0.9755282581475768211, 0.9755282581475770431, 1.000000000000000000, 0.9510565162951535312, 1.000000000000000000, 0.9510565162951569729, 0.9999999999999965583 ) ) 
 REPRESENTATION_ITEM ( '' )  );
#16419=DIRECTION ( 'NONE',  ( 0.000000000000000000, -1.000000000000000000, 0.000000000000000000 ) ) ;
#16437=CARTESIAN_POINT ( 'NONE',  ( 20.64299112944278036, 16.99999999999997868, 11.19067762888292350 ) ) ;
#16464=CARTESIAN_POINT ( 'NONE',  ( -7.570916362186210335, 14.60000000000000142, -23.30088464923126779 ) ) ;
#16467=CARTESIAN_POINT ( 'NONE',  ( -23.41746825000000243, 11.72499999726879949, 7.608796670333725309 ) ) ;
#16468=CARTESIAN_POINT ( 'NONE',  ( -19.82091636218621034, 8.800000000000002487, -14.40073868116559552 ) ) ;
#16471=CARTESIAN_POINT ( 'NONE',  ( 22.66806446082019733, 16.99999999999997868, -6.072923278005473158 ) ) ;
#16501=CARTESIAN_POINT ( 'NONE',  ( 1.507698388325705758E-15, 13.12499999726881228, -24.62258325217400312 ) ) ;
#16507=EDGE_CURVE ( 'NONE', #12563, #13367, #9620, .T. ) ;
#16523=CARTESIAN_POINT ( 'NONE',  ( -14.47279130897151589, 13.32499999726880624, -19.92008829642072598 ) ) ;
#16525=ORIENTED_EDGE ( 'NONE', *, *, #15453, .F. ) ;
#16537=CARTESIAN_POINT ( 'NONE',  ( -15.14183272437242778, 3.049999994537633263, 20.84094480462497856 ) ) ;
#16544=SURFACE_STYLE_FILL_AREA ( #19123 ) ;
#16549=VERTEX_POINT ( 'NONE', #21125 ) ;
#16550=CARTESIAN_POINT ( 'NONE',  ( -24.50000000000001066, 18.84999999453762953, 7.960532557706201828 ) ) ;
#16553=EDGE_CURVE ( 'NONE', #16741, #6266, #21717, .T. ) ;
#16567=CARTESIAN_POINT ( 'NONE',  ( 7.236395654485755280, 16.72499999726881370, 22.27133577429736988 ) ) ;
#16590=DIRECTION ( 'NONE',  ( 0.000000000000000000, 0.000000000000000000, -1.000000000000000000 ) ) ;
#16599=CARTESIAN_POINT ( 'NONE',  ( 15.26205751043174885, 16.99999999999997868, 18.11263815609570926 ) ) ;
#16620=CARTESIAN_POINT ( 'NONE',  ( 19.82091636218621389, 15.94999999453763984, -14.40073868116559197 ) ) ;
#16632=CARTESIAN_POINT ( 'NONE',  ( -4.732186688966233175E-15, 13.50000000000001066, 25.76082449383753925 ) ) ;
#16636=CARTESIAN_POINT ( 'NONE',  ( 23.41746824999999887, 12.72499999726882791, -7.608796670333727974 ) ) ;
#16642=CARTESIAN_POINT ( 'NONE',  ( 18.59695232317482905, 16.99999999999998224, -14.25184196307220219 ) ) ;
#16657=ORIENTED_EDGE ( 'NONE', *, *, #29829, .F. ) ;
#16670=CARTESIAN_POINT ( 'NONE',  ( -7.236395654485757944, 13.22499999726881015, -22.27133577429736988 ) ) ;
#16691=CARTESIAN_POINT ( 'NONE',  ( 18.94512977948576093, 16.82499999726880091, -13.76444248337722875 ) ) ;
#16696=CARTESIAN_POINT ( 'NONE',  ( -7.236395654485757944, 3.724999997268802154, -22.27133577429736988 ) ) ;
#16720=CARTESIAN_POINT ( 'NONE',  ( 14.47279130897151589, 8.824999997268804464, 19.92008829642072953 ) ) ;
#16735=CARTESIAN_POINT ( 'NONE',  ( 23.41746824999999887, 13.12499999726882116, 0.000000000000000000 ) ) ;
#16741=VERTEX_POINT ( 'NONE', #3759 ) ;
#16757=CARTESIAN_POINT ( 'NONE',  ( -7.570916362186210335, 16.34999999453762243, -23.30088464923126779 ) ) ;
#16764=CARTESIAN_POINT ( 'NONE',  ( 16.34000363327193384, 17.00000000000000000, 17.09839857644911731 ) ) ;
#16772=CARTESIAN_POINT ( 'NONE',  ( -15.14183272437242778, 11.04999999453761284, 20.84094480462497856 ) ) ;
#16801=CARTESIAN_POINT ( 'NONE',  ( -15.14183272437242600, 9.299999999999998934, 20.84094480462497856 ) ) ;
#16806=CARTESIAN_POINT ( 'NONE',  ( -7.236395654485757944, 9.224999997268806595, -22.27133577429736988 ) ) ;
#16807=CARTESIAN_POINT ( 'NONE',  ( -3.712076227271900841E-14, 8.499999999999994671, -24.50000000000000000 ) ) ;
#16815=DIRECTION ( 'NONE',  ( 0.000000000000000000, 0.000000000000000000, -1.000000000000000000 ) ) ;
#16824=EDGE_CURVE ( 'NONE', #14840, #16549, #2368, .T. ) ;
#16836=CARTESIAN_POINT ( 'NONE',  ( 3.880418787951172011, 11.55125428154683576, 24.49999999999998579 ) ) ;
#16840=CARTESIAN_POINT ( 'NONE',  ( 23.41746825000000243, 14.52499999726882685, 7.608796670333735079 ) ) ;
#16862=EDGE_LOOP ( 'NONE', ( #20121, #24868, #1751, #31959 ) ) ;
#16864=CARTESIAN_POINT ( 'NONE',  ( -14.47279130897152299, 2.424999997268802332, 19.92008829642072243 ) ) ;
#16877=( LENGTH_UNIT ( ) NAMED_UNIT ( * ) SI_UNIT ( .MILLI., .METRE. ) );
#16884=CARTESIAN_POINT ( 'NONE',  ( 23.41746825000000243, 5.224999997268802154, -7.608796670333727974 ) ) ;
#16900=CARTESIAN_POINT ( 'NONE',  ( 14.47279130897151767, 4.924999997268811214, -19.92008829642072598 ) ) ;
#16909=ORIENTED_EDGE ( 'NONE', *, *, #29977, .F. ) ;
#16915=EDGE_CURVE ( 'NONE', #19128, #6559, #17095, .T. ) ;
#16924=EDGE_CURVE ( 'NONE', #476, #14840, #14644, .T. ) ;
#16926=CARTESIAN_POINT ( 'NONE',  ( 19.82091636218621034, 7.549999994537620829, 14.40073868116559730 ) ) ;
#16933=CARTESIAN_POINT ( 'NONE',  ( -13.41233651847560182, 16.99999999999998934, 20.39142027516456679 ) ) ;
#16935=CARTESIAN_POINT ( 'NONE',  ( 19.82091636218621034, 1.799999999999996048, 14.40073868116559730 ) ) ;
#16936=( BOUNDED_CURVE ( )  B_SPLINE_CURVE ( 2, ( #16807, #14059, #11151, #24029, #16468, #8226, #24684, #27263, #29156, #18879, #19214, #29328, #32065 ),
 .UNSPECIFIED., .F., .F. ) 
 B_SPLINE_CURVE_WITH_KNOTS ( ( 3, 2, 2, 2, 2, 2, 3 ),
 ( 0.4722222222222222654, 0.4777777777777778012, 0.4888888888888888729, 0.5000000000000000000, 0.5111111111111110716, 0.5222222222222222543, 0.5277777777777777901 ),
 .UNSPECIFIED. ) 
 CURVE ( )  GEOMETRIC_REPRESENTATION_ITEM ( )  RATIONAL_B_SPLINE_CURVE ( ( 0.9755282581475767101, 0.9755282581475768211, 1.000000000000000000, 0.9510565162951535312, 1.000000000000000000, 0.9510565162951535312, 1.000000000000000000, 0.9510565162951535312, 1.000000000000000000, 0.9510565162951535312, 1.000000000000000000, 0.9755282581475768211, 0.9755282581475768211 ) ) 
 REPRESENTATION_ITEM ( '' )  );
#16943=CARTESIAN_POINT ( 'NONE',  ( -3.880418787951136483, 12.55125428154685174, -24.50000000000000000 ) ) ;
#16953=CARTESIAN_POINT ( 'NONE',  ( 7.570916362186213000, 16.14999999453761603, -23.30088464923126423 ) ) ;
#16967=CARTESIAN_POINT ( 'NONE',  ( -4.732186688966233175E-15, 11.49999999999998579, 25.76082449383753925 ) ) ;
#16971=CARTESIAN_POINT ( 'NONE',  ( 23.41746824999999887, 12.62499999726882116, 0.000000000000000000 ) ) ;
#16976=CARTESIAN_POINT ( 'NONE',  ( 15.46695104312588498, 16.99999999999998224, -17.59928039462594640 ) ) ;
#16993=( BOUNDED_CURVE ( )  B_SPLINE_CURVE ( 2, ( #19438, #21847, #27659, #19269, #4148, #6215, #19939, #29886, #12034, #30218, #25077, #32791, #19604, #16864, #14621, #17030, #32955, #27489, #3979, #11529, #1558, #24741, #11869, #11697, #22344, #9284, #16696, #27152, #19768, #24577, #6719, #1049, #14789, #890, #27325, #3813, #14285, #31082, #7578, #18057, #4828, #25603, #4487, #28502, #18231, #33485, #1728, #15139, #33659, #22853, #15308, #4999, #9986, #10330, #25767, #15482, #25936, #25253, #14963, #28677, #28000, #17713, #20806, #2253, #25429, #12208, #30910, #20459, #5174, #2082, #12897, #20117, #12557, #12727, #12384, #22679, #10157, #1907, #7404, #2429, #23028, #20639, #33130, #23197, #20287, #17890, #9634, #28343, #23372, #33833, #31250, #7742, #30561, #7058, #9810, #33311, #17540, #30734, #7227, #28171, #4659, #2939, #26107, #23878, #3, #5343, #32086, #10832, #28844, #23542, #2769, #21311, #13233, #2605, #8411, #10493, #18900, #20970, #683, #11169, #31752, #31421, #8243, #23707, #18736, #31919, #13066, #16161, #15824, #7914, #21640, #29346, #29178, #5683, #10663, #173, #26615, #13410, #24046, #5847, #18398, #8582, #3112, #26278, #21142, #31583, #13584, #8083, #18570, #16326, #29011, #26782, #5511, #19066, #29506, #515, #11002, #15657, #15992, #3273, #13741 ),
 .UNSPECIFIED., .F., .F. ) 
 B_SPLINE_CURVE_WITH_KNOTS ( ( 3, 2, 2, 2, 2, 2, 2, 2, 2, 2, 2, 2, 2, 2, 2, 2, 2, 2, 2, 2, 2, 2, 2, 2, 2, 2, 2, 2, 2, 2, 2, 2, 2, 2, 2, 2, 2, 2, 2, 2, 2, 2, 2, 2, 2, 2, 2, 2, 2, 2, 2, 2, 2, 2, 2, 2, 2, 2, 2, 2, 2, 2, 2, 2, 2, 2, 2, 2, 2, 2, 2, 2, 2, 2, 2, 2, 2, 2, 2, 2, 3 ),
 ( 0.000000000000000000, 0.01111111111111111154, 0.02222222222222222307, 0.03333333333333333287, 0.04444444444444444614, 0.05555555555555555247, 0.06666666666666666574, 0.07777777777777779289, 0.08888888888888889228, 0.1000000000000000056, 0.1111111111111111049, 0.1222222222222222182, 0.1333333333333333315, 0.1444444444444444309, 0.1555555555555555858, 0.1666666666666666574, 0.1777777777777777846, 0.1888888888888888840, 0.2000000000000000111, 0.2111111111111111105, 0.2222222222222222099, 0.2333333333333333370, 0.2444444444444444364, 0.2555555555555555358, 0.2666666666666666630, 0.2777777777777777901, 0.2888888888888888618, 0.2999999999999999889, 0.3111111111111111716, 0.3222222222222222432, 0.3333333333333333148, 0.3444444444444444420, 0.3555555555555555691, 0.3666666666666666408, 0.3777777777777777679, 0.3888888888888888951, 0.4000000000000000222, 0.4111111111111110938, 0.4222222222222222210, 0.4333333333333333481, 0.4444444444444444198, 0.4555555555555555469, 0.4666666666666666741, 0.4777777777777777457, 0.4888888888888888729, 0.5000000000000000000, 0.5111111111111110716, 0.5222222222222222543, 0.5333333333333333259, 0.5444444444444443976, 0.5555555555555555802, 0.5666666666666666519, 0.5777777777777777235, 0.5888888888888889062, 0.5999999999999999778, 0.6111111111111111605, 0.6222222222222223431, 0.6333333333333333037, 0.6444444444444444864, 0.6555555555555555580, 0.6666666666666666297, 0.6777777777777778123, 0.6888888888888888840, 0.6999999999999999556, 0.7111111111111111382, 0.7222222222222222099, 0.7333333333333332815, 0.7444444444444445752, 0.7555555555555555358, 0.7666666666666667185, 0.7777777777777777901, 0.7888888888888888618, 0.8000000000000000444, 0.8111111111111111160, 0.8222222222222221877, 0.8333333333333332593, 0.8444444444444444420, 0.8555555555555555136, 0.8666666666666666963, 0.8777777777777777679, 0.8819764054827600175 ),
 .UNSPECIFIED. ) 
 CURVE ( )  GEOMETRIC_REPRESENTATION_ITEM ( )  RATIONAL_B_SPLINE_CURVE ( ( 1.000000000000000000, 0.9510565162951535312, 1.000000000000000000, 0.9510565162951535312, 1.000000000000000000, 0.9510565162951535312, 1.000000000000000000, 0.9510565162951535312, 1.000000000000000000, 0.9510565162951535312, 1.000000000000000000, 0.9510565162951535312, 1.000000000000000000, 0.9510565162951535312, 1.000000000000000000, 0.9510565162951535312, 1.000000000000000000, 0.9510565162951535312, 1.000000000000000000, 0.9510565162951535312, 1.000000000000000000, 0.9510565162951535312, 1.000000000000000000, 0.9510565162951535312, 1.000000000000000000, 0.9510565162951535312, 1.000000000000000000, 0.9510565162951535312, 1.000000000000000000, 0.9510565162951535312, 1.000000000000000000, 0.9510565162951535312, 1.000000000000000000, 0.9510565162951535312, 1.000000000000000000, 0.9510565162951535312, 1.000000000000000000, 0.9510565162951535312, 1.000000000000000000, 0.9510565162951535312, 1.000000000000000000, 0.9510565162951535312, 1.000000000000000000, 0.9510565162951535312, 1.000000000000000000, 0.9510565162951535312, 1.000000000000000000, 0.9510565162951535312, 1.000000000000000000, 0.9510565162951535312, 1.000000000000000000, 0.9510565162951535312, 1.000000000000000000, 0.9510565162951535312, 1.000000000000000000, 0.9510565162951535312, 1.000000000000000000, 0.9510565162951535312, 1.000000000000000000, 0.9510565162951535312, 1.000000000000000000, 0.9510565162951535312, 1.000000000000000000, 0.9510565162951535312, 1.000000000000000000, 0.9510565162951535312, 1.000000000000000000, 0.9510565162951535312, 1.000000000000000000, 0.9510565162951535312, 1.000000000000000000, 0.9510565162951535312, 1.000000000000000000, 0.9510565162951535312, 1.000000000000000000, 0.9510565162951535312, 1.000000000000000000, 0.9510565162951535312, 1.000000000000000000, 0.9510565162951535312, 1.000000000000000000, 0.9510565162951535312, 1.000000000000000000, 0.9510565162951535312, 1.000000000000000000, 0.9510565162951535312, 1.000000000000000000, 0.9510565162951535312, 1.000000000000000000, 0.9510565162951535312, 1.000000000000000000, 0.9510565162951535312, 1.000000000000000000, 0.9510565162951535312, 1.000000000000000000, 0.9510565162951535312, 1.000000000000000000, 0.9510565162951535312, 1.000000000000000000, 0.9510565162951535312, 1.000000000000000000, 0.9510565162951535312, 1.000000000000000000, 0.9510565162951535312, 1.000000000000000000, 0.9510565162951535312, 1.000000000000000000, 0.9510565162951535312, 1.000000000000000000, 0.9510565162951535312, 1.000000000000000000, 0.9510565162951535312, 1.000000000000000000, 0.9510565162951535312, 1.000000000000000000, 0.9510565162951535312, 1.000000000000000000, 0.9510565162951535312, 1.000000000000000000, 0.9510565162951535312, 1.000000000000000000, 0.9510565162951535312, 1.000000000000000000, 0.9510565162951535312, 1.000000000000000000, 0.9510565162951535312, 1.000000000000000000, 0.9510565162951535312, 1.000000000000000000, 0.9510565162951535312, 1.000000000000000000, 0.9510565162951535312, 1.000000000000000000, 0.9510565162951535312, 1.000000000000000000, 0.9510565162951535312, 1.000000000000000000, 0.9510565162951535312, 1.000000000000000000, 0.9510565162951535312, 1.000000000000000000, 0.9510565162951535312, 1.000000000000000000, 0.9510565162951535312, 1.000000000000000000, 0.9510565162951535312, 1.000000000000000000, 0.9510565162951535312, 1.000000000000000000, 0.9510565162951535312, 1.000000000000000000, 0.9510565162951535312, 1.000000000000000000, 0.9510565162951535312, 1.000000000000000000, 0.9510565162951535312, 1.000000000000000000, 0.9510565162951535312, 1.000000000000000000, 0.9815054080004634862, 0.9769881591460145565 ) ) 
 REPRESENTATION_ITEM ( '' )  );
#17006=CARTESIAN_POINT ( 'NONE',  ( -23.41746825000000243, 11.52499999726880553, -7.608796670333730638 ) ) ;
#17030=CARTESIAN_POINT ( 'NONE',  ( -4.523095164977117273E-15, 2.624999997268825602, 24.62258325217400312 ) ) ;
#17051=CARTESIAN_POINT ( 'NONE',  ( -23.41746824999999887, 8.124999997268817609, -2.867812753649727150E-15 ) ) ;
#17060=ADVANCED_FACE ( 'NONE', ( #26055 ), #2716, .T. ) ;
#17067=CARTESIAN_POINT ( 'NONE',  ( 14.47279130897151589, 18.82499999726881157, 19.92008829642072953 ) ) ;
#17092=CARTESIAN_POINT ( 'NONE',  ( 19.82091636218621389, 7.949999994537631842, -14.40073868116559197 ) ) ;
#17095=( BOUNDED_CURVE ( )  B_SPLINE_CURVE ( 2, ( #4091, #7172, #15078, #22622, #17653, #24853, #28114, #2026, #17312, #12327, #1334, #33074, #1673 ),
 .UNSPECIFIED., .F., .T. ) 
 B_SPLINE_CURVE_WITH_KNOTS ( ( 3, 2, 2, 2, 2, 2, 3 ),
 ( 0.1388888888888888951, 0.1444444444444444309, 0.1555555555555555580, 0.1666666666666666574, 0.1777777777777777846, 0.1888888888888888840, 0.1944444444444444475 ),
 .UNSPECIFIED. ) 
 CURVE ( )  GEOMETRIC_REPRESENTATION_ITEM ( )  RATIONAL_B_SPLINE_CURVE ( ( 0.9755282581475768211, 0.9755282581475768211, 1.000000000000000000, 0.9510565162951535312, 1.000000000000000000, 0.9510565162951535312, 1.000000000000000000, 0.9510565162951535312, 1.000000000000000000, 0.9510565162951535312, 1.000000000000000000, 0.9755282581475768211, 0.9755282581475768211 ) ) 
 REPRESENTATION_ITEM ( '' )  );
#17103=CARTESIAN_POINT ( 'NONE',  ( 0.000000000000000000, 16.99999999999998579, -24.50000000000000000 ) ) ;
#17107=CARTESIAN_POINT ( 'NONE',  ( -14.47279130897152122, 4.424999997268826313, 19.92008829642072243 ) ) ;
#17114=ORIENTED_EDGE ( 'NONE', *, *, #33702, .T. ) ;
#17139=CARTESIAN_POINT ( 'NONE',  ( 15.14183272437242245, 16.30000000000001137, -20.84094480462497856 ) ) ;
#17143=CARTESIAN_POINT ( 'NONE',  ( -18.94512977948575738, 13.42499999726881654, -13.76444248337723231 ) ) ;
#17147=CARTESIAN_POINT ( 'NONE',  ( -23.09300878900790366, 16.99999999999999289, -7.697900481730200362 ) ) ;
#17177=CARTESIAN_POINT ( 'NONE',  ( 23.41746825000000243, 12.52499999726880375, 7.608796670333735079 ) ) ;
#17217=FILL_AREA_STYLE_COLOUR ( '', #20050 ) ;
#17220=CARTESIAN_POINT ( 'NONE',  ( 3.880418787951121828, 8.448745718453148257, -24.50000000000000355 ) ) ;
#17224=CARTESIAN_POINT ( 'NONE',  ( -7.236395654485763274, 4.524999997268825069, 22.27133577429736633 ) ) ;
#17236=CARTESIAN_POINT ( 'NONE',  ( -7.236395654485763274, 2.024999997268822405, 22.27133577429736633 ) ) ;
#17247=VERTEX_POINT ( 'NONE', #629 ) ;
#17260=CARTESIAN_POINT ( 'NONE',  ( -7.570916362186210335, 8.349999994537615322, -23.30088464923126779 ) ) ;
#17267=CARTESIAN_POINT ( 'NONE',  ( 0.000000000000000000, 16.99999999999998579, -24.50000000000000000 ) ) ;
#17268=CARTESIAN_POINT ( 'NONE',  ( 24.50000000000000000, 2.099999999999991651, -7.960532557706203605 ) ) ;
#17286=CARTESIAN_POINT ( 'NONE',  ( -15.14183272437242778, 3.300000000000012257, 20.84094480462497856 ) ) ;
#17312=CARTESIAN_POINT ( 'NONE',  ( -19.82091636218621389, 4.949999994537629178, 14.40073868116558842 ) ) ;
#17343=CARTESIAN_POINT ( 'NONE',  ( 24.50000000000000355, 2.099999999999991651, -7.960532557706203605 ) ) ;
#17369=EDGE_LOOP ( 'NONE', ( #2732, #18965, #30821, #15442 ) ) ;
#17384=CARTESIAN_POINT ( 'NONE',  ( -23.41746825000000598, 1.724999997268824581, 7.608796670333726198 ) ) ;
#17394=CARTESIAN_POINT ( 'NONE',  ( 1.507698388325705758E-15, 7.624999997268814056, -24.62258325217400312 ) ) ;
#17409=CARTESIAN_POINT ( 'NONE',  ( 14.47279130897151767, 0.9249999972688209837, -19.92008829642072598 ) ) ;
#17434=CARTESIAN_POINT ( 'NONE',  ( -24.50000000000000000, 6.749999994537625447, -3.000384657911015469E-15 ) ) ;
#17442=CARTESIAN_POINT ( 'NONE',  ( 3.880418787951139592, 1.551254281546846192, 24.50000000000000000 ) ) ;
#17450=FACE_OUTER_BOUND ( 'NONE', #11369, .T. ) ;
#17481=CARTESIAN_POINT ( 'NONE',  ( -23.41746825000000243, 15.72499999726882081, 7.608796670333725309 ) ) ;
#17485=CARTESIAN_POINT ( 'NONE',  ( -23.40419987650453848, 16.99999999999998579, -6.773127805312867622 ) ) ;
#17511=CARTESIAN_POINT ( 'NONE',  ( 3.880418787951172011, 13.30125427608447097, 24.49999999999998579 ) ) ;
#17515=CARTESIAN_POINT ( 'NONE',  ( -4.523095164977116484E-15, 16.12499999726880873, 24.62258325217400312 ) ) ;
#17536=EDGE_CURVE ( 'NONE', #13996, #24889, #3883, .T. ) ;
#17540=CARTESIAN_POINT ( 'NONE',  ( 7.236395654485755280, 10.72499999726880837, 22.27133577429736988 ) ) ;
#17541=ORIENTED_EDGE ( 'NONE', *, *, #17881, .T. ) ;
#17548=ORIENTED_EDGE ( 'NONE', *, *, #31693, .T. ) ;
#17557=FACE_OUTER_BOUND ( 'NONE', #8004, .T. ) ;
#17566=CARTESIAN_POINT ( 'NONE',  ( -18.94512977948576093, 16.32499999726880091, 13.76444248337722698 ) ) ;
#17579=CARTESIAN_POINT ( 'NONE',  ( -14.47279130897151589, 3.324999997268803131, -19.92008829642072598 ) ) ;
#17588=ORIENTED_EDGE ( 'NONE', *, *, #9209, .T. ) ;
#17601=CARTESIAN_POINT ( 'NONE',  ( 19.82091636218621034, 13.54999999453762527, 14.40073868116559730 ) ) ;
#17608=LINE ( 'NONE', #17267, #2411 ) ;
#17645=CARTESIAN_POINT ( 'NONE',  ( -19.82091636218621034, 16.80000000000000782, -14.40073868116559552 ) ) ;
#17650=CARTESIAN_POINT ( 'NONE',  ( -4.523095164977117273E-15, 14.12499999726881050, 24.62258325217400312 ) ) ;
#17653=CARTESIAN_POINT ( 'NONE',  ( -19.82091636218621034, 4.549999994537618164, -14.40073868116559552 ) ) ;
#17682=( LENGTH_UNIT ( ) NAMED_UNIT ( * ) SI_UNIT ( .MILLI., .METRE. ) );
#17687=CARTESIAN_POINT ( 'NONE',  ( -23.41746825000000598, 17.72499999726881725, 7.608796670333726198 ) ) ;
#17703=CARTESIAN_POINT ( 'NONE',  ( 3.880418787951140036, 6.448745718453147369, -24.49999999999999645 ) ) ;
#17713=CARTESIAN_POINT ( 'NONE',  ( 23.41746824999999887, 7.224999997268826135, -7.608796670333727974 ) ) ;
#17734=CARTESIAN_POINT ( 'NONE',  ( 24.50000000000000000, 7.900000000000012790, 7.960532557706212486 ) ) ;
#17736=ORIENTED_EDGE ( 'NONE', *, *, #31186, .F. ) ;
#17737=CARTESIAN_POINT ( 'NONE',  ( -18.94512977948575738, 13.92499999726881654, -13.76444248337723231 ) ) ;
#17738=CARTESIAN_POINT ( 'NONE',  ( 23.41746824999999887, 4.524999997268823293, 7.608796670333735079 ) ) ;
#17751=CARTESIAN_POINT ( 'NONE',  ( -7.236395654485763274, 10.02499999726880198, 22.27133577429736633 ) ) ;
#17776=CARTESIAN_POINT ( 'NONE',  ( 24.50000000000000355, 15.84999999453763664, -7.960532557706203605 ) ) ;
#17789=CARTESIAN_POINT ( 'NONE',  ( -18.94512977948576093, 4.324999997268818674, 13.76444248337722698 ) ) ;
#17796=VERTEX_POINT ( 'NONE', #28917 ) ;
#17810=CARTESIAN_POINT ( 'NONE',  ( -3.880418787951124493, 5.448745718453149145, 24.50000000000000355 ) ) ;
#17828=CARTESIAN_POINT ( 'NONE',  ( -10.07379044330640028, 16.99999999999998579, -21.64901441059538101 ) ) ;
#17832=LINE ( 'NONE', #23139, #32517 ) ;
#17863=CARTESIAN_POINT ( 'NONE',  ( -7.236395654485757944, 15.22499999726881192, -22.27133577429736988 ) ) ;
#17865=FACE_BOUND ( 'NONE', #22510, .T. ) ;
#17878=CARTESIAN_POINT ( 'NONE',  ( 3.445340210940985210E-14, 5.499999999999997335, 24.50000000000000000 ) ) ;
#17881=EDGE_CURVE ( 'NONE', #17796, #12037, #3064, .T. ) ;
#17890=CARTESIAN_POINT ( 'NONE',  ( 1.507698388325705758E-15, 9.624999997268808727, -24.62258325217400312 ) ) ;
#17891=ORIENTED_EDGE ( 'NONE', *, *, #16553, .F. ) ;
#17898=CARTESIAN_POINT ( 'NONE',  ( 7.570916362186213000, 6.149999994537635573, -23.30088464923126423 ) ) ;
#17916=CARTESIAN_POINT ( 'NONE',  ( 23.41746825000000243, 11.02499999726882152, 7.608796670333735079 ) ) ;
#17917=CARTESIAN_POINT ( 'NONE',  ( 7.236395654485760609, 3.024999997268823293, -22.27133577429736633 ) ) ;
#17919=( BOUNDED_CURVE ( )  B_SPLINE_CURVE ( 2, ( #1618, #10224, #33726, #15372, #20004, #25662, #33017, #20703, #33546, #12268, #12096, #20346, #25827 ),
 .UNSPECIFIED., .F., .F. ) 
 B_SPLINE_CURVE_WITH_KNOTS ( ( 3, 2, 2, 2, 2, 2, 3 ),
 ( 0.6944444444444444198, 0.6999999999999999556, 0.7111111111111111382, 0.7222222222222222099, 0.7333333333333332815, 0.7444444444444444642, 0.7500000000000000000 ),
 .UNSPECIFIED. ) 
 CURVE ( )  GEOMETRIC_REPRESENTATION_ITEM ( )  RATIONAL_B_SPLINE_CURVE ( ( 0.9755282581475768211, 0.9755282581475768211, 1.000000000000000000, 0.9510565162951535312, 1.000000000000000000, 0.9510565162951535312, 1.000000000000000000, 0.9510565162951535312, 1.000000000000000000, 0.9510565162951535312, 1.000000000000000000, 0.9755282581475768211, 0.9755282581475768211 ) ) 
 REPRESENTATION_ITEM ( '' )  );
#17931=CARTESIAN_POINT ( 'NONE',  ( 23.41746825000000243, 6.724999997268811924, -7.608796670333727974 ) ) ;
#17932=CARTESIAN_POINT ( 'NONE',  ( 3.880418787951134707, 13.55125428154684997, 24.50000000000000000 ) ) ;
#17955=CARTESIAN_POINT ( 'NONE',  ( 19.82091636218621389, 11.94999999453763628, -14.40073868116559197 ) ) ;
#17962=CARTESIAN_POINT ( 'NONE',  ( -15.14183272437242778, 7.300000000000001599, 20.84094480462497856 ) ) ;
#17968=CARTESIAN_POINT ( 'NONE',  ( -14.47279130897151589, 9.824999997268802687, -19.92008829642072598 ) ) ;
#17980=CARTESIAN_POINT ( 'NONE',  ( -3.880418787951146697, 2.551254281546845526, -24.49999999999999645 ) ) ;
#18003=CARTESIAN_POINT ( 'NONE',  ( -14.47279130897152299, 15.92499999726881121, 19.92008829642072243 ) ) ;
#18026=CARTESIAN_POINT ( 'NONE',  ( 0.000000000000000000, 16.99999999999998579, 0.000000000000000000 ) ) ;
#18036=CARTESIAN_POINT ( 'NONE',  ( -7.570916362186215665, 1.400000000000012346, 23.30088464923126423 ) ) ;
#18049=CARTESIAN_POINT ( 'NONE',  ( 3.880418787951172011, 15.55125428154684819, 24.49999999999998579 ) ) ;
#18057=CARTESIAN_POINT ( 'NONE',  ( 23.41746824999999887, 5.024999997268808194, 7.608796670333735079 ) ) ;
#18082=CARTESIAN_POINT ( 'NONE',  ( -23.41746824999999887, 12.12499999726882116, -2.867812753649727150E-15 ) ) ;
#18083=CARTESIAN_POINT ( 'NONE',  ( 7.236395654485760609, 1.024999997268821739, -22.27133577429736633 ) ) ;
#18095=CARTESIAN_POINT ( 'NONE',  ( 18.94512977948576093, 8.824999997268822227, -13.76444248337722875 ) ) ;
#18116=CARTESIAN_POINT ( 'NONE',  ( 7.313012447739250820E-14, 15.50000000000000178, 24.50000000000000000 ) ) ;
#18123=CARTESIAN_POINT ( 'NONE',  ( 15.14183272437241889, 13.44999999453762385, 20.84094480462498211 ) ) ;
#18139=CARTESIAN_POINT ( 'NONE',  ( 18.94512977948575738, 8.924999997268812990, 13.76444248337723408 ) ) ;
#18147=ORIENTED_EDGE ( 'NONE', *, *, #6732, .T. ) ;
#18207=CARTESIAN_POINT ( 'NONE',  ( -19.82091636218621389, 5.200000000000009948, 14.40073868116558842 ) ) ;
#18231=CARTESIAN_POINT ( 'NONE',  ( 7.236395654485760609, 5.524999997268825958, -22.27133577429736633 ) ) ;
#18247=CARTESIAN_POINT ( 'NONE',  ( 23.41746825000000243, 2.724999997268822138, -7.608796670333727974 ) ) ;
#18257=CARTESIAN_POINT ( 'NONE',  ( -23.41746825000000598, 16.22499999726880304, 7.608796670333726198 ) ) ;
#18268=CARTESIAN_POINT ( 'NONE',  ( -14.47279130897152122, 7.924999997268803220, 19.92008829642072243 ) ) ;
#18277=EDGE_CURVE ( 'NONE', #14369, #21231, #8963, .T. ) ;
#18286=CARTESIAN_POINT ( 'NONE',  ( -3.880418787951124493, 7.198745712990782586, 24.50000000000000355 ) ) ;
#18296=CARTESIAN_POINT ( 'NONE',  ( -19.82091636218621389, 14.94999999453763806, 14.40073868116558842 ) ) ;
#18311=CARTESIAN_POINT ( 'NONE',  ( -14.47279130897151589, 5.824999997268811569, -19.92008829642072598 ) ) ;
#18321=CARTESIAN_POINT ( 'NONE',  ( 15.14183272437242422, 10.29999999999999361, -20.84094480462497856 ) ) ;
#18334=LINE ( 'NONE', #28605, #20667 ) ;
#18350=CARTESIAN_POINT ( 'NONE',  ( -19.82091636218621034, 12.54999999453762527, -14.40073868116559552 ) ) ;
#18376=CARTESIAN_POINT ( 'NONE',  ( 7.570916362186213000, 2.400000000000013234, -23.30088464923126423 ) ) ;
#18383=CARTESIAN_POINT ( 'NONE',  ( 19.82091636218621389, 9.949999994537634507, -14.40073868116559197 ) ) ;
#18387=LINE ( 'NONE', #28833, #19922 ) ;
#18392=DIRECTION ( 'NONE',  ( 0.000000000000000000, 0.000000000000000000, -1.000000000000000000 ) ) ;
#18398=CARTESIAN_POINT ( 'NONE',  ( 23.41746824999999887, 15.12499999726882294, 0.000000000000000000 ) ) ;
#18402=EDGE_CURVE ( 'NONE', #23373, #28296, #12480, .T. ) ;
#18409=DIRECTION ( 'NONE',  ( 0.000000000000000000, -1.000000000000000000, 0.000000000000000000 ) ) ;
#18417=CARTESIAN_POINT ( 'NONE',  ( 18.94512977948576093, 2.824999997268817786, -13.76444248337722875 ) ) ;
#18430=AXIS2_PLACEMENT_3D ( 'NONE', #5790, #9188, #5957 ) ;
#18440=CARTESIAN_POINT ( 'NONE',  ( 18.94512977948575738, 8.424999997268811214, 13.76444248337723408 ) ) ;
#18454=CARTESIAN_POINT ( 'NONE',  ( -1.756012107511856980E-14, 6.249999994537623671, -24.50000000000000000 ) ) ;
#18463=CARTESIAN_POINT ( 'NONE',  ( 19.82091636218621034, 17.54999999453762882, 14.40073868116559730 ) ) ;
#18478=CARTESIAN_POINT ( 'NONE',  ( -23.41746825000000243, 6.024999997268805529, -7.608796670333730638 ) ) ;
#18488=LINE ( 'NONE', #10116, #24719 ) ;
#18503=CARTESIAN_POINT ( 'NONE',  ( -3.880418787951136483, 16.30125427608446742, -24.50000000000000000 ) ) ;
#18543=CARTESIAN_POINT ( 'NONE',  ( -4.732186688966233175E-15, 3.500000000000005329, 25.76082449383753925 ) ) ;
#18570=CARTESIAN_POINT ( 'NONE',  ( -18.94512977948575738, 15.92499999726881832, -13.76444248337723231 ) ) ;
#18586=CARTESIAN_POINT ( 'NONE',  ( 1.507698388325705758E-15, 7.124999997268828267, -24.62258325217400312 ) ) ;
#18608=CARTESIAN_POINT ( 'NONE',  ( -7.236395654485757944, 17.22499999726881370, -22.27133577429736988 ) ) ;
#18610=CARTESIAN_POINT ( 'NONE',  ( 1.555960095263670572E-15, 14.50000000000000178, -24.50000000000000000 ) ) ;
#18622=CARTESIAN_POINT ( 'NONE',  ( 6.001560367445586717E-15, 3.249999994537631665, 24.50000000000000000 ) ) ;
#18636=CARTESIAN_POINT ( 'NONE',  ( -7.570916362186215665, 17.14999999453761959, 23.30088464923126423 ) ) ;
#18649=CARTESIAN_POINT ( 'NONE',  ( -23.41746825000000598, 8.224999997268824359, 7.608796670333726198 ) ) ;
#18660=CARTESIAN_POINT ( 'NONE',  ( 3.000384657911015469E-15, 16.99999999999998579, 24.50000000000000000 ) ) ;
#18685=CARTESIAN_POINT ( 'NONE',  ( -7.579748464070165821E-14, 12.24999999453762456, -24.50000000000000000 ) ) ;
#18714=CARTESIAN_POINT ( 'NONE',  ( 19.82091636218621389, 6.200000000000010836, -14.40073868116559197 ) ) ;
#18719=CARTESIAN_POINT ( 'NONE',  ( 23.41746824999999887, 2.624999997268812280, 0.000000000000000000 ) ) ;
#18720=CARTESIAN_POINT ( 'NONE',  ( -1.756012107511856980E-14, 4.249999994537631665, -24.50000000000000000 ) ) ;
#18724=CARTESIAN_POINT ( 'NONE',  ( 24.50000000000000000, 1.749999994537621006, 0.000000000000000000 ) ) ;
#18736=CARTESIAN_POINT ( 'NONE',  ( 7.236395654485760609, 13.52499999726880553, -22.27133577429736633 ) ) ;
#18752=CARTESIAN_POINT ( 'NONE',  ( 23.41746825000000243, 4.724999997268818142, -7.608796670333727974 ) ) ;
#18772=CARTESIAN_POINT ( 'NONE',  ( 18.94512977948576093, 14.82499999726880091, -13.76444248337722875 ) ) ;
#18783=CIRCLE ( 'NONE', #16042, 24.50000000000000000 ) ;
#18798=CARTESIAN_POINT ( 'NONE',  ( 24.50000000000000355, 17.64999999453763380, 7.960532557706212486 ) ) ;
#18807=DIRECTION ( 'NONE',  ( 0.000000000000000000, 0.000000000000000000, -1.000000000000000000 ) ) ;
#18812=VECTOR ( 'NONE', #96, 1000.000000000000000 ) ;
#18813=CARTESIAN_POINT ( 'NONE',  ( -14.47279130897152122, 12.42499999726880766, 19.92008829642072243 ) ) ;
#18821=CARTESIAN_POINT ( 'NONE',  ( -7.570916362186215665, 1.400000000000012346, 23.30088464923126423 ) ) ;
#18853=DIRECTION ( 'NONE',  ( 0.000000000000000000, 0.000000000000000000, -1.000000000000000000 ) ) ;
#18873=CARTESIAN_POINT ( 'NONE',  ( -15.14183272437241889, 12.70000000000000639, -20.84094480462497856 ) ) ;
#18875=CARTESIAN_POINT ( 'NONE',  ( 15.14183272437241889, 5.449999994537614079, 20.84094480462498211 ) ) ;
#18878=CARTESIAN_POINT ( 'NONE',  ( 23.41746824999999887, 6.624999997268815832, 0.000000000000000000 ) ) ;
#18879=CARTESIAN_POINT ( 'NONE',  ( -15.14183272437242778, 9.299999999999995381, 20.84094480462497856 ) ) ;
#18883=CARTESIAN_POINT ( 'NONE',  ( 20.29802760220268709, 16.99999999999999289, -11.70263796218577745 ) ) ;
#18900=CARTESIAN_POINT ( 'NONE',  ( 7.236395654485755280, 12.72499999726881015, 22.27133577429736988 ) ) ;
#18917=CARTESIAN_POINT ( 'NONE',  ( 7.236395654485755280, 6.224999997268803931, 22.27133577429736988 ) ) ;
#18925=CARTESIAN_POINT ( 'NONE',  ( 23.41746824999999887, 19.12499999726882649, 0.000000000000000000 ) ) ;
#18941=CARTESIAN_POINT ( 'NONE',  ( 23.41746825000000243, 12.72499999726882436, -7.608796670333727974 ) ) ;
#18942=CARTESIAN_POINT ( 'NONE',  ( 15.14183272437242422, 14.30000000000001492, -20.84094480462497856 ) ) ;
#18956=FACE_OUTER_BOUND ( 'NONE', #8267, .T. ) ;
#18965=ORIENTED_EDGE ( 'NONE', *, *, #5376, .T. ) ;
#18966=CARTESIAN_POINT ( 'NONE',  ( 1.577395562988744260E-15, 16.24999999453762456, -25.76082449383753925 ) ) ;
#18980=CARTESIAN_POINT ( 'NONE',  ( -7.236395654485757944, 13.72499999726881015, -22.27133577429736988 ) ) ;
#19012=CARTESIAN_POINT ( 'NONE',  ( 18.29076905308899370, 16.99999999999997868, 14.90902754751065906 ) ) ;
#19045=CARTESIAN_POINT ( 'NONE',  ( 7.570916362186213000, 14.39999999999999680, -23.30088464923126423 ) ) ;
#19048=CARTESIAN_POINT ( 'NONE',  ( 18.94512977948576093, 12.82499999726882578, -13.76444248337722875 ) ) ;
#19049=CARTESIAN_POINT ( 'NONE',  ( 19.82091636218621034, 3.799999999999998046, 14.40073868116559730 ) ) ;
#19066=CARTESIAN_POINT ( 'NONE',  ( -14.47279130897152299, 16.42499999726882720, 19.92008829642072243 ) ) ;
#19080=CARTESIAN_POINT ( 'NONE',  ( 23.41746824999999887, 10.62499999726881938, 0.000000000000000000 ) ) ;
#19089=CARTESIAN_POINT ( 'NONE',  ( 0.000000000000000000, 16.99999999999998579, 0.000000000000000000 ) ) ;
#19102=CARTESIAN_POINT ( 'NONE',  ( -7.236395654485763274, 16.02499999726880731, 22.27133577429736633 ) ) ;
#19113=EDGE_CURVE ( 'NONE', #14205, #19228, #18783, .T. ) ;
#19123=FILL_AREA_STYLE ('',( #17217 ) ) ;
#19128=VERTEX_POINT ( 'NONE', #20064 ) ;
#19129=CARTESIAN_POINT ( 'NONE',  ( -4.732186688966233175E-15, 19.24999999453761745, 25.76082449383753925 ) ) ;
#19144=CARTESIAN_POINT ( 'NONE',  ( -7.236395654485763274, 16.52499999726880731, 22.27133577429736633 ) ) ;
#19157=DIRECTION ( 'NONE',  ( 0.000000000000000000, 0.000000000000000000, -1.000000000000000000 ) ) ;
#19177=CARTESIAN_POINT ( 'NONE',  ( -15.82193040522741967, 16.99999999999999645, 18.67333929100095347 ) ) ;
#19183=CYLINDRICAL_SURFACE ( 'NONE', #29695, 26.50000000000000355 ) ;
#19185=CARTESIAN_POINT ( 'NONE',  ( 1.555960095263670572E-15, 12.50000000000000355, -24.50000000000000000 ) ) ;
#19207=CARTESIAN_POINT ( 'NONE',  ( -24.50000000000000000, 11.00000000000001066, -3.000384657911015469E-15 ) ) ;
#19212=CARTESIAN_POINT ( 'NONE',  ( -14.47279130897151767, 9.324999997268816898, -19.92008829642072598 ) ) ;
#19214=CARTESIAN_POINT ( 'NONE',  ( -7.570916362186215665, 9.399999999999991473, 23.30088464923126423 ) ) ;
#19228=VERTEX_POINT ( 'NONE', #7694 ) ;
#19244=CARTESIAN_POINT ( 'NONE',  ( 23.41746824999999887, 12.62499999726882116, 0.000000000000000000 ) ) ;
#19251=VERTEX_POINT ( 'NONE', #15943 ) ;
#19265=CARTESIAN_POINT ( 'NONE',  ( 14.47279130897151589, 14.32499999726880624, 19.92008829642072953 ) ) ;
#19269=CARTESIAN_POINT ( 'NONE',  ( 14.47279130897151944, 1.424999997268804997, -19.92008829642072598 ) ) ;
#19291=CARTESIAN_POINT ( 'NONE',  ( -18.94512977948576093, 6.324999997268820451, 13.76444248337722698 ) ) ;
#19309=CARTESIAN_POINT ( 'NONE',  ( 18.94512977948576093, 13.32499999726879913, -13.76444248337722875 ) ) ;
#19317=CARTESIAN_POINT ( 'NONE',  ( -3.880418787951138260, 1.448745718453166020, 24.50000000000000000 ) ) ;
#19331=CARTESIAN_POINT ( 'NONE',  ( -19.82091636218621034, 16.54999999453762882, -14.40073868116559552 ) ) ;
#19343=( BOUNDED_CURVE ( )  B_SPLINE_CURVE ( 2, ( #498, #8896, #13726, #19380, #29826, #6330, #3754, #14228, #1159, #11640, #31898, #31735, #18720 ),
 .UNSPECIFIED., .F., .T. ) 
 B_SPLINE_CURVE_WITH_KNOTS ( ( 3, 2, 2, 2, 2, 2, 3 ),
 ( 0.08333333333333334259, 0.08888888888888889228, 0.1000000000000000056, 0.1111111111111111049, 0.1222222222222222321, 0.1333333333333333315, 0.1388888888888888951 ),
 .UNSPECIFIED. ) 
 CURVE ( )  GEOMETRIC_REPRESENTATION_ITEM ( )  RATIONAL_B_SPLINE_CURVE ( ( 0.9755282581475768211, 0.9755282581475768211, 1.000000000000000000, 0.9510565162951535312, 1.000000000000000000, 0.9510565162951535312, 1.000000000000000000, 0.9510565162951535312, 1.000000000000000000, 0.9510565162951535312, 1.000000000000000000, 0.9755282581475767101, 0.9755282581475768211 ) ) 
 REPRESENTATION_ITEM ( '' )  );
#19356=VERTEX_POINT ( 'NONE', #15429 ) ;
#19375=CARTESIAN_POINT ( 'NONE',  ( 24.50000000000000355, 11.90000000000000391, 7.960532557706212486 ) ) ;
#19379=CARTESIAN_POINT ( 'NONE',  ( -14.47279130897152299, 9.924999997268827201, 19.92008829642072243 ) ) ;
#19380=CARTESIAN_POINT ( 'NONE',  ( 15.14183272437242067, 3.449999994537619852, 20.84094480462498211 ) ) ;
#19412=CARTESIAN_POINT ( 'NONE',  ( -18.94512977948576093, 13.82499999726879913, 13.76444248337722698 ) ) ;
#19422=LINE ( 'NONE', #1378, #28332 ) ;
#19434=EDGE_CURVE ( 'NONE', #24093, #14205, #28795, .T. ) ;
#19438=CARTESIAN_POINT ( 'NONE',  ( 23.41746824999999887, 1.124999997268810725, 0.000000000000000000 ) ) ;
#19460=ORIENTED_EDGE ( 'NONE', *, *, #20163, .F. ) ;
#19461=CARTESIAN_POINT ( 'NONE',  ( 7.236395654485755280, 6.724999997268804819, 22.27133577429736988 ) ) ;
#19475=CARTESIAN_POINT ( 'NONE',  ( -4.523095164977116484E-15, 14.62499999726882649, 24.62258325217400312 ) ) ;
#19500=CARTESIAN_POINT ( 'NONE',  ( 24.50000000000000355, 5.649999994537638237, 7.960532557706212486 ) ) ;
#19508=CARTESIAN_POINT ( 'NONE',  ( 2.535219702907248518, 16.99999999999999289, 23.89400104877895714 ) ) ;
#19526=CARTESIAN_POINT ( 'NONE',  ( 3.880418787951134707, 15.30125427608446742, 24.50000000000000000 ) ) ;
#19539=ADVANCED_FACE ( 'NONE', ( #3725 ), #19183, .T. ) ;
#19542=CARTESIAN_POINT ( 'NONE',  ( -24.50000000000001066, 11.09999999999999964, 7.960532557706201828 ) ) ;
#19546=CARTESIAN_POINT ( 'NONE',  ( 23.41746824999999887, 8.524999997268812635, 7.608796670333735079 ) ) ;
#19550=CARTESIAN_POINT ( 'NONE',  ( 14.28720042100528609, 16.99999999999998579, -18.56979130494320529 ) ) ;
#19554=CARTESIAN_POINT ( 'NONE',  ( 1.555960095263670572E-15, 14.50000000000000178, -24.50000000000000000 ) ) ;
#19576=CARTESIAN_POINT ( 'NONE',  ( 7.570916362186213000, 12.39999999999999503, -23.30088464923126423 ) ) ;
#19580=CARTESIAN_POINT ( 'NONE',  ( -23.41746824999999887, 11.62499999726881938, -2.867812753649727150E-15 ) ) ;
#19604=CARTESIAN_POINT ( 'NONE',  ( -18.94512977948576093, 2.324999997268817342, 13.76444248337722698 ) ) ;
#19616=AXIS2_PLACEMENT_3D ( 'NONE', #28071, #9533, #22252 ) ;
#19625=ORIENTED_EDGE ( 'NONE', *, *, #22429, .T. ) ;
#19626=CARTESIAN_POINT ( 'NONE',  ( -23.41746824999999887, 10.12499999726881938, -2.867812753649727150E-15 ) ) ;
#19636=CARTESIAN_POINT ( 'NONE',  ( 7.570916362186213000, 16.39999999999999858, -23.30088464923126423 ) ) ;
#19641=CARTESIAN_POINT ( 'NONE',  ( -23.41746824999999887, 3.624999997268813168, -2.867812753649727150E-15 ) ) ;
#19651=ORIENTED_EDGE ( 'NONE', *, *, #16090, .T. ) ;
#19665=CARTESIAN_POINT ( 'NONE',  ( -24.50000000000001066, 4.849999994537633974, 7.960532557706201828 ) ) ;
#19672=CARTESIAN_POINT ( 'NONE',  ( 19.94128806827436406, 16.99999999999997868, 12.49245821715489946 ) ) ;
#19679=CARTESIAN_POINT ( 'NONE',  ( -18.94512977948575738, 1.924999997268805885, -13.76444248337723231 ) ) ;
#19710=CARTESIAN_POINT ( 'NONE',  ( 7.236395654485760609, 13.02499999726880375, -22.27133577429736633 ) ) ;
#19714=CARTESIAN_POINT ( 'NONE',  ( -11.85439961466680359, 16.99999999999997868, -20.79774841451609291 ) ) ;
#19722=EDGE_CURVE ( 'NONE', #6266, #33508, #30709, .T. ) ;
#19745=CARTESIAN_POINT ( 'NONE',  ( -14.47279130897152122, 11.92499999726882010, 19.92008829642072243 ) ) ;
#19768=CARTESIAN_POINT ( 'NONE',  ( -18.94512977948575738, 3.924999997268807661, -13.76444248337723231 ) ) ;
#19789=CARTESIAN_POINT ( 'NONE',  ( 7.236395654485755280, 4.724999997268803043, 22.27133577429736988 ) ) ;
#19805=CARTESIAN_POINT ( 'NONE',  ( 7.236395654485760609, 5.024999997268825069, -22.27133577429736633 ) ) ;
#19828=CARTESIAN_POINT ( 'NONE',  ( 15.14183272437242245, 8.049999994537621717, -20.84094480462497856 ) ) ;
#19841=CARTESIAN_POINT ( 'NONE',  ( 18.94512977948576093, 5.324999997268820451, -13.76444248337722875 ) ) ;
#19843=ADVANCED_FACE ( 'NONE', ( #17450 ), #2673, .T. ) ;
#19844=DIRECTION ( 'NONE',  ( 0.000000000000000000, 0.000000000000000000, -1.000000000000000000 ) ) ;
#19854=CARTESIAN_POINT ( 'NONE',  ( -1.756012107511856980E-14, 2.500000000000005773, -24.50000000000000000 ) ) ;
#19872=CARTESIAN_POINT ( 'NONE',  ( 15.14183272437241889, 17.69999999999999218, 20.84094480462498211 ) ) ;
#19880=CARTESIAN_POINT ( 'NONE',  ( -17.34916400531743363, 16.99999999999998579, -16.72523852671361766 ) ) ;
#19881=LINE ( 'NONE', #30334, #7818 ) ;
#19914=CARTESIAN_POINT ( 'NONE',  ( -19.82091636218621389, 1.200000000000006617, 14.40073868116558842 ) ) ;
#19922=VECTOR ( 'NONE', #28665, 1000.000000000000000 ) ;
#19939=CARTESIAN_POINT ( 'NONE',  ( -7.236395654485757944, 1.724999997268800156, -22.27133577429736988 ) ) ;
#19957=CARTESIAN_POINT ( 'NONE',  ( -7.236395654485757944, 1.224999997268799712, -22.27133577429736988 ) ) ;
#19967=CARTESIAN_POINT ( 'NONE',  ( -18.94512977948575738, 3.924999997268807661, -13.76444248337723231 ) ) ;
#19980=CARTESIAN_POINT ( 'NONE',  ( 7.236395654485755280, 2.224999997268800378, 22.27133577429736988 ) ) ;
#20004=CARTESIAN_POINT ( 'NONE',  ( -19.82091636218621034, 14.54999999453762705, -14.40073868116559552 ) ) ;
#20006=CARTESIAN_POINT ( 'NONE',  ( 24.50000000000000355, 5.849999994537631309, -7.960532557706203605 ) ) ;
#20020=CARTESIAN_POINT ( 'NONE',  ( 23.41746824999999887, 1.124999997268810725, 0.000000000000000000 ) ) ;
#20032=CARTESIAN_POINT ( 'NONE',  ( 3.445340210940985210E-14, 9.249999994537636994, 24.50000000000000000 ) ) ;
#20050=COLOUR_RGB ( '', 0.31764706, 0.68627451, 0.89019608) ;
#20064=CARTESIAN_POINT ( 'NONE',  ( -1.756012107511856980E-14, 4.249999994537631665, -24.50000000000000000 ) ) ;
#20091=CARTESIAN_POINT ( 'NONE',  ( 1.507698388325705758E-15, 17.12499999726880517, -24.62258325217400312 ) ) ;
#20117=CARTESIAN_POINT ( 'NONE',  ( -23.41746825000000243, 8.224999997268822582, 7.608796670333725309 ) ) ;
#20121=ORIENTED_EDGE ( 'NONE', *, *, #18277, .F. ) ;
#20134=DIRECTION ( 'NONE',  ( 0.000000000000000000, 0.000000000000000000, -1.000000000000000000 ) ) ;
#20142=CARTESIAN_POINT ( 'NONE',  ( 23.41746825000000243, 15.02499999726881086, 7.608796670333735079 ) ) ;
#20155=CARTESIAN_POINT ( 'NONE',  ( 14.47279130897151589, 2.324999997268805796, 19.92008829642072953 ) ) ;
#20163=EDGE_CURVE ( 'NONE', #14665, #9893, #245, .T. ) ;
#20179=CARTESIAN_POINT ( 'NONE',  ( -7.570916362186215665, 15.14999999453761603, 23.30088464923126423 ) ) ;
#20188=CARTESIAN_POINT ( 'NONE',  ( 15.14183272437242422, 2.299999999999985612, -20.84094480462497856 ) ) ;
#20189=VECTOR ( 'NONE', #5627, 1000.000000000000000 ) ;
#20230=CARTESIAN_POINT ( 'NONE',  ( 23.41746824999999887, 16.72499999726881725, -7.608796670333727974 ) ) ;
#20234=CARTESIAN_POINT ( 'NONE',  ( -12.70562935223222034, 16.99999999999998934, -20.31534774774085150 ) ) ;
#20259=CARTESIAN_POINT ( 'NONE',  ( 15.14183272437242067, 13.44999999453762385, 20.84094480462498211 ) ) ;
#20263=CARTESIAN_POINT ( 'NONE',  ( -23.41746824999999887, 15.62499999726882294, -2.867812753649727150E-15 ) ) ;
#20282=CARTESIAN_POINT ( 'NONE',  ( 24.50000000000000000, 0.000000000000000000, 0.000000000000000000 ) ) ;
#20287=CARTESIAN_POINT ( 'NONE',  ( 7.236395654485760609, 9.524999997268828622, -22.27133577429736633 ) ) ;
#20307=( BOUNDED_CURVE ( )  B_SPLINE_CURVE ( 2, ( #3058, #29457, #3718, #24158, #8194, #24644, #11118, #13859, #11603, #8529, #21586, #22085, #18685 ),
 .UNSPECIFIED., .F., .T. ) 
 B_SPLINE_CURVE_WITH_KNOTS ( ( 3, 2, 2, 2, 2, 2, 3 ),
 ( 0.5277777777777777901, 0.5333333333333333259, 0.5444444444444443976, 0.5555555555555555802, 0.5666666666666666519, 0.5777777777777777235, 0.5833333333333333703 ),
 .UNSPECIFIED. ) 
 CURVE ( )  GEOMETRIC_REPRESENTATION_ITEM ( )  RATIONAL_B_SPLINE_CURVE ( ( 0.9755282581475768211, 0.9755282581475768211, 1.000000000000000000, 0.9510565162951535312, 1.000000000000000000, 0.9510565162951535312, 1.000000000000000000, 0.9510565162951535312, 1.000000000000000000, 0.9510565162951535312, 1.000000000000000000, 0.9755282581475765991, 0.9755282581475768211 ) ) 
 REPRESENTATION_ITEM ( '' )  );
#20310=CARTESIAN_POINT ( 'NONE',  ( -7.236395654485763274, 12.52499999726880375, 22.27133577429736633 ) ) ;
#20311=CARTESIAN_POINT ( 'NONE',  ( -7.236395654485757944, 3.224999997268801266, -22.27133577429736988 ) ) ;
#20325=CARTESIAN_POINT ( 'NONE',  ( 18.94512977948576093, 10.82499999726882578, -13.76444248337722875 ) ) ;
#20346=CARTESIAN_POINT ( 'NONE',  ( -3.880418787951142701, 15.19874571299077282, 24.49999999999999645 ) ) ;
#20348=CARTESIAN_POINT ( 'NONE',  ( -7.570916362186215665, 11.14999999453761248, 23.30088464923126423 ) ) ;
#20364=CARTESIAN_POINT ( 'NONE',  ( -23.41746824999999887, 2.124999997268811391, -2.867812753649727150E-15 ) ) ;
#20392=CARTESIAN_POINT ( 'NONE',  ( -15.14183272437242600, 15.30000000000001137, 20.84094480462497856 ) ) ;
#20398=CARTESIAN_POINT ( 'NONE',  ( 23.41746824999999887, 14.72499999726882081, -7.608796670333727974 ) ) ;
#20400=CARTESIAN_POINT ( 'NONE',  ( -22.54140686924021963, 16.99999999999999645, -9.059062350126763974 ) ) ;
#20433=CARTESIAN_POINT ( 'NONE',  ( 19.82091636218621389, 0.2000000000000057288, -14.40073868116559197 ) ) ;
#20449=CARTESIAN_POINT ( 'NONE',  ( 7.313012447739250820E-14, 15.50000000000000178, 24.50000000000000000 ) ) ;
#20459=CARTESIAN_POINT ( 'NONE',  ( -14.47279130897151767, 7.824999997268806240, -19.92008829642072598 ) ) ;
#20467=CARTESIAN_POINT ( 'NONE',  ( -1.756012107511856980E-14, 6.249999994537623671, -24.50000000000000000 ) ) ;
#20484=ORIENTED_EDGE ( 'NONE', *, *, #20914, .T. ) ;
#20485=CARTESIAN_POINT ( 'NONE',  ( -4.523095164977116484E-15, 12.62499999726879985, 24.62258325217400312 ) ) ;
#20486=CARTESIAN_POINT ( 'NONE',  ( -23.41746824999999887, 3.524999997268825958, -7.608796670333730638 ) ) ;
#20501=CARTESIAN_POINT ( 'NONE',  ( 14.47279130897151767, 10.92499999726882365, -19.92008829642072598 ) ) ;
#20530=CARTESIAN_POINT ( 'NONE',  ( -19.82091636218621389, 12.94999999453763628, 14.40073868116558842 ) ) ;
#20543=CARTESIAN_POINT ( 'NONE',  ( 23.41746825000000243, 11.22499999726881548, -7.608796670333727974 ) ) ;
#20599=ORIENTED_EDGE ( 'NONE', *, *, #3020, .T. ) ;
#20615=CARTESIAN_POINT ( 'NONE',  ( 19.82091636218621034, 1.799999999999996048, 14.40073868116559730 ) ) ;
#20625=CARTESIAN_POINT ( 'NONE',  ( -3.712076227271900841E-14, 10.24999999453763344, -24.50000000000000000 ) ) ;
#20639=CARTESIAN_POINT ( 'NONE',  ( 23.41746824999999887, 9.224999997268820806, -7.608796670333727974 ) ) ;
#20667=VECTOR ( 'NONE', #2706, 1000.000000000000000 ) ;
#20668=CARTESIAN_POINT ( 'NONE',  ( 7.236395654485760609, 11.52499999726880375, -22.27133577429736633 ) ) ;
#20669=CARTESIAN_POINT ( 'NONE',  ( 14.47279130897151767, 2.324999997268806240, 19.92008829642072953 ) ) ;
#20682=CARTESIAN_POINT ( 'NONE',  ( -23.41746824999999887, 7.624999997268816720, -2.867812753649727150E-15 ) ) ;
#20684=ORIENTED_EDGE ( 'NONE', *, *, #7884, .F. ) ;
#20703=CARTESIAN_POINT ( 'NONE',  ( -24.50000000000000711, 14.84999999453763841, 7.960532557706201828 ) ) ;
#20704=EDGE_CURVE ( 'NONE', #24126, #12037, #23888, .T. ) ;
#20706=CARTESIAN_POINT ( 'NONE',  ( -24.50000000000000355, 12.64999999453762136, -7.960532557706207157 ) ) ;
#20714=ADVANCED_FACE ( 'NONE', ( #15668, #26118 ), #13078, .T. ) ;
#20720=CARTESIAN_POINT ( 'NONE',  ( 1.507698388325705758E-15, 11.62499999726880340, -24.62258325217400312 ) ) ;
#20765=ORIENTED_EDGE ( 'NONE', *, *, #12073, .T. ) ;
#20772=PLANE ( 'NONE',  #10828 ) ;
#20783=CARTESIAN_POINT ( 'NONE',  ( -19.82091636218621034, 6.800000000000000711, -14.40073868116559552 ) ) ;
#20792=CARTESIAN_POINT ( 'NONE',  ( 15.14183272437242422, 10.04999999453761639, -20.84094480462497856 ) ) ;
#20802=CARTESIAN_POINT ( 'NONE',  ( 15.14183272437242422, 0.2999999999999904965, -20.84094480462497856 ) ) ;
#20806=CARTESIAN_POINT ( 'NONE',  ( 18.94512977948576093, 7.324999997268822227, -13.76444248337722875 ) ) ;
#20816=CARTESIAN_POINT ( 'NONE',  ( 0.000000000000000000, 16.99999999999998579, -15.00000000000000000 ) ) ;
#20822=CARTESIAN_POINT ( 'NONE',  ( 14.47279130897151767, 2.924999997268815655, -19.92008829642072598 ) ) ;
#20832=CARTESIAN_POINT ( 'NONE',  ( -14.47279130897151589, 15.82499999726881335, -19.92008829642072598 ) ) ;
#20843=CARTESIAN_POINT ( 'NONE',  ( 1.507698388325705758E-15, 9.124999997268822938, -24.62258325217400312 ) ) ;
#20844=CARTESIAN_POINT ( 'NONE',  ( 19.82091636218621389, 14.19999999999999041, -14.40073868116559197 ) ) ;
#20867=CARTESIAN_POINT ( 'NONE',  ( -19.82091636218621034, 14.54999999453762705, -14.40073868116559552 ) ) ;
#20882=CARTESIAN_POINT ( 'NONE',  ( 23.41746825000000243, 7.224999997268826135, -7.608796670333727974 ) ) ;
#20914=EDGE_CURVE ( 'NONE', #26574, #6391, #7057, .T. ) ;
#20929=ORIENTED_EDGE ( 'NONE', *, *, #24795, .F. ) ;
#20948=CARTESIAN_POINT ( 'NONE',  ( -4.732186688966233175E-15, 5.500000000000000888, 25.76082449383753925 ) ) ;
#20950=CARTESIAN_POINT ( 'NONE',  ( -19.82091636218621034, 2.549999994537616388, -14.40073868116559552 ) ) ;
#20956=CARTESIAN_POINT ( 'NONE',  ( 3.445340210940985210E-14, 9.249999994537636994, 24.50000000000000000 ) ) ;
#20970=CARTESIAN_POINT ( 'NONE',  ( 14.47279130897151767, 12.82499999726882400, 19.92008829642072953 ) ) ;
#20980=CARTESIAN_POINT ( 'NONE',  ( 15.14183272437242422, 6.049999994537626158, -20.84094480462497856 ) ) ;
#20988=CARTESIAN_POINT ( 'NONE',  ( -18.94512977948575738, 3.424999997268807217, -13.76444248337723231 ) ) ;
#21010=CARTESIAN_POINT ( 'NONE',  ( 23.41746825000000243, 10.52499999726880731, 7.608796670333735079 ) ) ;
#21037=CARTESIAN_POINT ( 'NONE',  ( -7.570916362186210335, 16.34999999453762243, -23.30088464923126779 ) ) ;
#21044=CARTESIAN_POINT ( 'NONE',  ( 1.555960095263670572E-15, 14.24999999453762278, -24.50000000000000000 ) ) ;
#21052=CARTESIAN_POINT ( 'NONE',  ( 14.47279130897151767, 9.424999997268814766, -19.92008829642072598 ) ) ;
#21058=ORIENTED_EDGE ( 'NONE', *, *, #33397, .T. ) ;
#21089=EDGE_CURVE ( 'NONE', #33874, #24889, #21512, .T. ) ;
#21090=CARTESIAN_POINT ( 'NONE',  ( 3.828750298241973660, 16.99999999999997868, -23.23455841446276082 ) ) ;
#21102=VERTEX_POINT ( 'NONE', #30703 ) ;
#21117=CARTESIAN_POINT ( 'NONE',  ( 7.570916362186207671, 3.599999999999992095, 23.30088464923126779 ) ) ;
#21125=CARTESIAN_POINT ( 'NONE',  ( 21.64573397815488676, 16.99999999999998579, 8.935324268693841887 ) ) ;
#21128=DIRECTION ( 'NONE',  ( 0.000000000000000000, 0.000000000000000000, 1.000000000000000000 ) ) ;
#21129=CARTESIAN_POINT ( 'NONE',  ( 0.000000000000000000, 16.99999999999998579, 0.000000000000000000 ) ) ;
#21142=CARTESIAN_POINT ( 'NONE',  ( 7.236395654485760609, 15.52499999726880731, -22.27133577429736633 ) ) ;
#21157=COLOUR_RGB ( '', 0.31764706, 0.68627451, 0.89019608) ;
#21159=CARTESIAN_POINT ( 'NONE',  ( -23.41746824999999887, 3.624999997268813168, -2.867812753649727150E-15 ) ) ;
#21170=AXIS2_PLACEMENT_3D ( 'NONE', #12225, #33150, #20134 ) ;
#21181=CARTESIAN_POINT ( 'NONE',  ( -7.236395654485763274, 18.02499999726880731, 22.27133577429736633 ) ) ;
#21205=CARTESIAN_POINT ( 'NONE',  ( 18.94512977948575738, 2.924999997268806773, 13.76444248337723408 ) ) ;
#21221=CARTESIAN_POINT ( 'NONE',  ( 7.236395654485760609, 7.524999997268827734, -22.27133577429736633 ) ) ;
#21231=VERTEX_POINT ( 'NONE', #10804 ) ;
#21258=CARTESIAN_POINT ( 'NONE',  ( -4.480168651474261132, 16.99999999999998579, -23.39706153295998448 ) ) ;
#21278=DIRECTION ( 'NONE',  ( 0.000000000000000000, -1.000000000000000000, 0.000000000000000000 ) ) ;
#21289=CARTESIAN_POINT ( 'NONE',  ( -19.82091636218621034, 4.799999999999998934, -14.40073868116559552 ) ) ;
#21294=CARTESIAN_POINT ( 'NONE',  ( 14.47279130897151767, 4.324999997268800911, 19.92008829642072953 ) ) ;
#21311=CARTESIAN_POINT ( 'NONE',  ( -23.41746825000000243, 12.22499999726881370, 7.608796670333725309 ) ) ;
#21326=CARTESIAN_POINT ( 'NONE',  ( -18.94512977948576093, 3.824999997268818674, 13.76444248337722698 ) ) ;
#21348=CARTESIAN_POINT ( 'NONE',  ( -4.523095164977116484E-15, 14.12499999726881050, 24.62258325217400312 ) ) ;
#21359=CARTESIAN_POINT ( 'NONE',  ( -24.50000000000000000, 2.749999994537621895, -3.000384657911015469E-15 ) ) ;
#21363=CARTESIAN_POINT ( 'NONE',  ( -19.82091636218621389, 6.949999994537630954, 14.40073868116558842 ) ) ;
#21367=CARTESIAN_POINT ( 'NONE',  ( -15.14183272437242778, 15.30000000000001137, 20.84094480462497856 ) ) ;
#21372=CARTESIAN_POINT ( 'NONE',  ( 1.577395562988744260E-15, 18.24999999453762101, -25.76082449383753925 ) ) ;
#21385=CARTESIAN_POINT ( 'NONE',  ( 1.507698388325705758E-15, 17.62499999726881938, -24.62258325217400312 ) ) ;
#21393=CARTESIAN_POINT ( 'NONE',  ( -15.14183272437242067, 0.7000000000000070610, -20.84094480462497856 ) ) ;
#21439=DIRECTION ( 'NONE',  ( 0.000000000000000000, 0.000000000000000000, -1.000000000000000000 ) ) ;
#21449=CARTESIAN_POINT ( 'NONE',  ( 19.82091636218621389, 4.200000000000009059, -14.40073868116559197 ) ) ;
#21454=CARTESIAN_POINT ( 'NONE',  ( -18.94512977948576093, 5.824999997268820451, 13.76444248337722698 ) ) ;
#21461=VECTOR ( 'NONE', #21742, 1000.000000000000000 ) ;
#21488=CARTESIAN_POINT ( 'NONE',  ( 7.236395654485755280, 8.224999997268806595, 22.27133577429736988 ) ) ;
#21508=CARTESIAN_POINT ( 'NONE',  ( -23.41746825000000243, 15.52499999726882507, -7.608796670333730638 ) ) ;
#21509=CARTESIAN_POINT ( 'NONE',  ( 7.570916362186213000, 14.39999999999999680, -23.30088464923126423 ) ) ;
#21512=( BOUNDED_CURVE ( )  B_SPLINE_CURVE ( 2, ( #7028, #17511, #25572, #20259, #28310, #1875, #33281, #7374, #12353, #22822, #9777, #4798, #15277 ),
 .UNSPECIFIED., .F., .T. ) 
 B_SPLINE_CURVE_WITH_KNOTS ( ( 3, 2, 2, 2, 2, 2, 3 ),
 ( 0.6388888888888889506, 0.6444444444444444864, 0.6555555555555555580, 0.6666666666666666297, 0.6777777777777778123, 0.6888888888888888840, 0.6944444444444444198 ),
 .UNSPECIFIED. ) 
 CURVE ( )  GEOMETRIC_REPRESENTATION_ITEM ( )  RATIONAL_B_SPLINE_CURVE ( ( 0.9755282581475768211, 0.9755282581475770431, 1.000000000000000000, 0.9510565162951535312, 1.000000000000000000, 0.9510565162951535312, 1.000000000000000000, 0.9510565162951535312, 1.000000000000000000, 0.9510565162951535312, 1.000000000000000000, 0.9755282581475768211, 0.9755282581475768211 ) ) 
 REPRESENTATION_ITEM ( '' )  );
#21520=VECTOR ( 'NONE', #28623, 1000.000000000000000 ) ;
#21525=DIRECTION ( 'NONE',  ( 0.000000000000000000, -1.000000000000000000, 0.000000000000000000 ) ) ;
#21528=LINE ( 'NONE', #15879, #16003 ) ;
#21534=CARTESIAN_POINT ( 'NONE',  ( 15.14183272437241889, 19.44999999453763806, 20.84094480462498211 ) ) ;
#21551=CARTESIAN_POINT ( 'NONE',  ( -23.41746825000000598, 18.22499999726882436, 7.608796670333726198 ) ) ;
#21561=CARTESIAN_POINT ( 'NONE',  ( -7.570916362186210335, 0.5999999999999894307, -23.30088464923126779 ) ) ;
#21565=CARTESIAN_POINT ( 'NONE',  ( 0.000000000000000000, 16.99999999999998579, 0.000000000000000000 ) ) ;
#21577=CARTESIAN_POINT ( 'NONE',  ( -7.570916362186215665, 11.39999999999999325, 23.30088464923126423 ) ) ;
#21584=CARTESIAN_POINT ( 'NONE',  ( 21.27620594755971695, 16.99999999999997868, 9.851211979822984688 ) ) ;
#21586=CARTESIAN_POINT ( 'NONE',  ( 7.570916362186213000, 12.14999999453761426, -23.30088464923126423 ) ) ;
#21604=CARTESIAN_POINT ( 'NONE',  ( 7.570916362186207671, 15.34999999453762243, 23.30088464923126779 ) ) ;
#21616=CARTESIAN_POINT ( 'NONE',  ( -7.570916362186215665, 13.39999999999999503, 23.30088464923126423 ) ) ;
#21621=CARTESIAN_POINT ( 'NONE',  ( 1.507698388325705758E-15, 11.12499999726881761, -24.62258325217400312 ) ) ;
#21622=CARTESIAN_POINT ( 'NONE',  ( 24.50000000000000000, 3.899999999999992806, 7.960532557706212486 ) ) ;
#21626=CARTESIAN_POINT ( 'NONE',  ( -6.668400408272875007E-16, 2.249999994537632553, -24.50000000000000355 ) ) ;
#21640=CARTESIAN_POINT ( 'NONE',  ( -23.41746824999999887, 14.12499999726882294, -2.867812753649727150E-15 ) ) ;
#21648=CARTESIAN_POINT ( 'NONE',  ( -7.579748464070167083E-14, 16.50000000000000355, -24.50000000000000000 ) ) ;
#21654=CARTESIAN_POINT ( 'NONE',  ( -14.47279130897152122, 9.924999997268825425, 19.92008829642072243 ) ) ;
#21662=CARTESIAN_POINT ( 'NONE',  ( 23.41746825000000243, 17.22499999726880304, -7.608796670333727974 ) ) ;
#21676=CARTESIAN_POINT ( 'NONE',  ( -4.523095164977116484E-15, 16.12499999726880873, 24.62258325217400312 ) ) ;
#21705=CARTESIAN_POINT ( 'NONE',  ( 18.94512977948576093, 3.324999997268818230, -13.76444248337722875 ) ) ;
#21717=( BOUNDED_CURVE ( )  B_SPLINE_CURVE ( 2, ( #20956, #26432, #13394, #23692, #8229, #2924, #2751, #4986, #18383, #20792, #28829, #5496, #20625 ),
 .UNSPECIFIED., .F., .T. ) 
 B_SPLINE_CURVE_WITH_KNOTS ( ( 3, 2, 2, 2, 2, 2, 3 ),
 ( 0.4166666666666666852, 0.4222222222222222210, 0.4333333333333333481, 0.4444444444444444198, 0.4555555555555555469, 0.4666666666666666741, 0.4722222222222222654 ),
 .UNSPECIFIED. ) 
 CURVE ( )  GEOMETRIC_REPRESENTATION_ITEM ( )  RATIONAL_B_SPLINE_CURVE ( ( 0.9755282581475767101, 0.9755282581475768211, 1.000000000000000000, 0.9510565162951535312, 1.000000000000000000, 0.9510565162951535312, 1.000000000000000000, 0.9510565162951535312, 1.000000000000000000, 0.9510565162951535312, 1.000000000000000000, 0.9755282581475765991, 0.9755282581475767101 ) ) 
 REPRESENTATION_ITEM ( '' )  );
#21722=CARTESIAN_POINT ( 'NONE',  ( 18.94512977948576093, 15.32499999726880091, -13.76444248337722875 ) ) ;
#21729=EDGE_LOOP ( 'NONE', ( #16657, #8325, #13283, #28007 ) ) ;
#21742=DIRECTION ( 'NONE',  ( 0.000000000000000000, -1.000000000000000000, 0.000000000000000000 ) ) ;
#21785=CARTESIAN_POINT ( 'NONE',  ( -7.570916362186210335, 10.59999999999999787, -23.30088464923126779 ) ) ;
#21788=CARTESIAN_POINT ( 'NONE',  ( -7.236395654485763274, 12.02499999726880375, 22.27133577429736633 ) ) ;
#21789=CARTESIAN_POINT ( 'NONE',  ( 7.570916362186207671, 3.599999999999992095, 23.30088464923126779 ) ) ;
#21802=AXIS2_PLACEMENT_3D ( 'NONE', #24588, #24424, #6397 ) ;
#21809=( BOUNDED_CURVE ( )  B_SPLINE_CURVE ( 2, ( #18454, #5227, #23594, #25991, #2658, #23427, #28897, #10889, #21363, #10379, #31806, #18286, #13289 ),
 .UNSPECIFIED., .F., .F. ) 
 B_SPLINE_CURVE_WITH_KNOTS ( ( 3, 2, 2, 2, 2, 2, 3 ),
 ( 0.2500000000000000000, 0.2555555555555555358, 0.2666666666666666630, 0.2777777777777777901, 0.2888888888888888618, 0.2999999999999999889, 0.3055555555555555802 ),
 .UNSPECIFIED. ) 
 CURVE ( )  GEOMETRIC_REPRESENTATION_ITEM ( )  RATIONAL_B_SPLINE_CURVE ( ( 0.9755282581475768211, 0.9755282581475768211, 1.000000000000000000, 0.9510565162951535312, 1.000000000000000000, 0.9510565162951535312, 1.000000000000000000, 0.9510565162951535312, 1.000000000000000000, 0.9510565162951535312, 1.000000000000000000, 0.9755282581475765991, 0.9755282581475767101 ) ) 
 REPRESENTATION_ITEM ( '' )  );
#21818=DIRECTION ( 'NONE',  ( 1.000000000000000000, 0.000000000000000000, 0.000000000000000000 ) ) ;
#21820=CARTESIAN_POINT ( 'NONE',  ( -4.523095164977116484E-15, 14.12499999726881050, 24.62258325217400312 ) ) ;
#21843=CARTESIAN_POINT ( 'NONE',  ( -18.94512977948576093, 13.82499999726879913, 13.76444248337722698 ) ) ;
#21847=CARTESIAN_POINT ( 'NONE',  ( 23.41746824999999887, 1.224999997268811480, -7.608796670333727974 ) ) ;
#21867=CARTESIAN_POINT ( 'NONE',  ( 23.41746824999999887, 7.124999997268815832, 0.000000000000000000 ) ) ;
#21882=CARTESIAN_POINT ( 'NONE',  ( 23.41746825000000243, 17.02499999726880731, 7.608796670333735079 ) ) ;
#21890=CARTESIAN_POINT ( 'NONE',  ( -24.50000000000000000, 1.000000000000000888, -3.000384657911015469E-15 ) ) ;
#21905=CARTESIAN_POINT ( 'NONE',  ( -7.570916362186210335, 10.59999999999999787, -23.30088464923126779 ) ) ;
#21913=CARTESIAN_POINT ( 'NONE',  ( 21.64573397815488676, 16.99999999999998579, 8.935324268693841887 ) ) ;
#21920=CARTESIAN_POINT ( 'NONE',  ( -24.50000000000000000, 10.64999999453762669, -7.960532557706207157 ) ) ;
#21922=CARTESIAN_POINT ( 'NONE',  ( -4.223320258572819786E-15, 13.50000000000000355, 24.50000000000000000 ) ) ;
#21945=CARTESIAN_POINT ( 'NONE',  ( -24.50000000000000000, 15.00000000000001421, -3.000384657911015469E-15 ) ) ;
#21949=CARTESIAN_POINT ( 'NONE',  ( -23.41746824999999887, 11.52499999726880553, -7.608796670333730638 ) ) ;
#21967=ORIENTED_EDGE ( 'NONE', *, *, #9886, .F. ) ;
#21985=CARTESIAN_POINT ( 'NONE',  ( -7.236395654485757944, 11.22499999726880837, -22.27133577429736988 ) ) ;
#21992=ORIENTED_EDGE ( 'NONE', *, *, #31174, .T. ) ;
#22034=CARTESIAN_POINT ( 'NONE',  ( -7.236395654485757944, 9.724999997268806595, -22.27133577429736988 ) ) ;
#22044=CARTESIAN_POINT ( 'NONE',  ( 24.50000000000000000, 16.09999999999998721, -7.960532557706203605 ) ) ;
#22047=CARTESIAN_POINT ( 'NONE',  ( 3.880418787951140036, 8.198745712990779921, -24.49999999999999645 ) ) ;
#22049=CARTESIAN_POINT ( 'NONE',  ( -23.41746824999999887, 12.12499999726882116, -2.867812753649727150E-15 ) ) ;
#22074=CARTESIAN_POINT ( 'NONE',  ( -19.82091636218621389, 8.949999994537632730, 14.40073868116558842 ) ) ;
#22082=CARTESIAN_POINT ( 'NONE',  ( 8.195098264072058214, 16.99999999999998934, 22.42925254762998932 ) ) ;
#22085=CARTESIAN_POINT ( 'NONE',  ( 3.880418787951102289, 12.19874571299077637, -24.50000000000000711 ) ) ;
#22103=CARTESIAN_POINT ( 'NONE',  ( -4.223320258572819786E-15, 15.24999999453762278, 24.50000000000000000 ) ) ;
#22118=CARTESIAN_POINT ( 'NONE',  ( -24.50000000000001066, 9.100000000000004974, 7.960532557706201828 ) ) ;
#22123=CARTESIAN_POINT ( 'NONE',  ( 18.94512977948575738, 12.42499999726881477, 13.76444248337723408 ) ) ;
#22127=CARTESIAN_POINT ( 'NONE',  ( 10.39950962648949684, 16.99999999999998579, -20.99551648793040926 ) ) ;
#22151=CARTESIAN_POINT ( 'NONE',  ( 15.14183272437242422, 12.29999999999999183, -20.84094480462497856 ) ) ;
#22157=CARTESIAN_POINT ( 'NONE',  ( 18.94512977948575738, 14.42499999726881654, 13.76444248337723408 ) ) ;
#22202=CARTESIAN_POINT ( 'NONE',  ( -18.94512977948575738, 7.924999997268811214, -13.76444248337723231 ) ) ;
#22211=CARTESIAN_POINT ( 'NONE',  ( 3.880418787951153803, 5.551254281546845526, 24.49999999999999645 ) ) ;
#22216=CARTESIAN_POINT ( 'NONE',  ( 18.94512977948576093, 4.824999997268819563, -13.76444248337722875 ) ) ;
#22241=CARTESIAN_POINT ( 'NONE',  ( 15.14183272437242245, 6.049999994537625270, -20.84094480462497856 ) ) ;
#22252=DIRECTION ( 'NONE',  ( 0.000000000000000000, 0.000000000000000000, -1.000000000000000000 ) ) ;
#22257=CARTESIAN_POINT ( 'NONE',  ( -23.41746824999999887, 4.124999997268813168, -2.867812753649727150E-15 ) ) ;
#22284=CARTESIAN_POINT ( 'NONE',  ( 7.570916362186213000, 12.39999999999999503, -23.30088464923126423 ) ) ;
#22288=CARTESIAN_POINT ( 'NONE',  ( 23.41746824999999887, 8.724999997268806595, -7.608796670333727974 ) ) ;
#22292=CARTESIAN_POINT ( 'NONE',  ( -21.91832052488144456, 17.00000000000000355, -10.39831318017644080 ) ) ;
#22322=CARTESIAN_POINT ( 'NONE',  ( -7.236395654485757944, 9.224999997268806595, -22.27133577429736988 ) ) ;
#22342=VERTEX_POINT ( 'NONE', #6105 ) ;
#22344=CARTESIAN_POINT ( 'NONE',  ( 7.236395654485760609, 3.524999997268824181, -22.27133577429736633 ) ) ;
#22365=CARTESIAN_POINT ( 'NONE',  ( 18.94512977948575738, 8.924999997268812990, 13.76444248337723408 ) ) ;
#22379=CARTESIAN_POINT ( 'NONE',  ( 7.236395654485755280, 4.224999997268802154, 22.27133577429736988 ) ) ;
#22402=CARTESIAN_POINT ( 'NONE',  ( 24.50000000000000355, 7.849999994537626868, -7.960532557706203605 ) ) ;
#22410=CARTESIAN_POINT ( 'NONE',  ( 0.000000000000000000, 16.99999999999998579, 0.000000000000000000 ) ) ;
#22415=CARTESIAN_POINT ( 'NONE',  ( 7.236395654485755280, 4.724999997268803043, 22.27133577429736988 ) ) ;
#22429=EDGE_CURVE ( 'NONE', #19356, #10883, #8514, .T. ) ;
#22460=ORIENTED_EDGE ( 'NONE', *, *, #24344, .F. ) ;
#22481=CARTESIAN_POINT ( 'NONE',  ( -7.236395654485757944, 17.22499999726881370, -22.27133577429736988 ) ) ;
#22510=EDGE_LOOP ( 'NONE', ( #31377, #29223 ) ) ;
#22529=CARTESIAN_POINT ( 'NONE',  ( 23.41746825000000243, 9.224999997268820806, -7.608796670333727974 ) ) ;
#22531=AXIS2_PLACEMENT_3D ( 'NONE', #10503, #18409, #5353 ) ;
#22542=CARTESIAN_POINT ( 'NONE',  ( -7.236395654485763274, 6.024999997268825958, 22.27133577429736633 ) ) ;
#22569=CARTESIAN_POINT ( 'NONE',  ( 15.14183272437241889, 9.449999994537636283, 20.84094480462498211 ) ) ;
#22583=CARTESIAN_POINT ( 'NONE',  ( 14.47279130897151767, 3.424999997268800112, -19.92008829642072598 ) ) ;
#22622=CARTESIAN_POINT ( 'NONE',  ( -15.14183272437242067, 4.449999994537617631, -20.84094480462497856 ) ) ;
#22653=CARTESIAN_POINT ( 'NONE',  ( 18.94512977948576093, 14.82499999726880091, -13.76444248337722875 ) ) ;
#22679=CARTESIAN_POINT ( 'NONE',  ( -4.523095164977117273E-15, 8.624999997268810503, 24.62258325217400312 ) ) ;
#22701=CARTESIAN_POINT ( 'NONE',  ( -3.712076227271900841E-14, 8.499999999999994671, -24.50000000000000000 ) ) ;
#22706=CARTESIAN_POINT ( 'NONE',  ( -14.47279130897152122, 14.42499999726880056, 19.92008829642072243 ) ) ;
#22723=CARTESIAN_POINT ( 'NONE',  ( -23.41746824999999887, 1.624999997268811169, -2.867812753649727150E-15 ) ) ;
#22745=CARTESIAN_POINT ( 'NONE',  ( -24.50000000000000000, 4.749999994537623671, -3.000384657911015469E-15 ) ) ;
#22759=CARTESIAN_POINT ( 'NONE',  ( 23.41746825000000243, 5.224999997268802154, -7.608796670333727974 ) ) ;
#22793=CARTESIAN_POINT ( 'NONE',  ( -7.236395654485757944, 15.22499999726881192, -22.27133577429736988 ) ) ;
#22797=CARTESIAN_POINT ( 'NONE',  ( -20.49854233591107189, 16.99999999999998579, -12.98872394473008463 ) ) ;
#22817=DIRECTION ( 'NONE',  ( 0.000000000000000000, -1.000000000000000000, 0.000000000000000000 ) ) ;
#22822=CARTESIAN_POINT ( 'NONE',  ( 15.14183272437242422, 14.04999999453763593, -20.84094480462497856 ) ) ;
#22826=CARTESIAN_POINT ( 'NONE',  ( 23.41746824999999887, 18.62499999726882649, 0.000000000000000000 ) ) ;
#22853=CARTESIAN_POINT ( 'NONE',  ( -23.41746824999999887, 6.024999997268805529, -7.608796670333730638 ) ) ;
#22864=ADVANCED_FACE ( 'NONE', ( #17557 ), #31819, .T. ) ;
#22879=CARTESIAN_POINT ( 'NONE',  ( 1.507698388325705758E-15, 15.62499999726882116, -24.62258325217400312 ) ) ;
#22893=CARTESIAN_POINT ( 'NONE',  ( -4.523095164977116484E-15, 4.124999997268806951, 24.62258325217400312 ) ) ;
#22919=CARTESIAN_POINT ( 'NONE',  ( -19.82091636218621034, 12.54999999453762527, -14.40073868116559552 ) ) ;
#22932=CARTESIAN_POINT ( 'NONE',  ( -7.236395654485763274, 2.524999997268823293, 22.27133577429736633 ) ) ;
#22945=CARTESIAN_POINT ( 'NONE',  ( 3.245314017740486554E-15, -20.99999999999998934, 26.50000000000000355 ) ) ;
#22960=CARTESIAN_POINT ( 'NONE',  ( 7.570916362186207671, 17.60000000000000497, 23.30088464923126779 ) ) ;
#23001=CARTESIAN_POINT ( 'NONE',  ( 23.41746825000000243, 18.52499999726881441, 7.608796670333735079 ) ) ;
#23009=DIRECTION ( 'NONE',  ( 0.000000000000000000, -1.000000000000000000, 0.000000000000000000 ) ) ;
#23015=CARTESIAN_POINT ( 'NONE',  ( 23.95873412499999944, 0.3124999986344190184, 0.000000000000000000 ) ) ;
#23022=CARTESIAN_POINT ( 'NONE',  ( 7.570916362186213000, 8.149999994537637349, -23.30088464923126423 ) ) ;
#23028=CARTESIAN_POINT ( 'NONE',  ( 23.41746824999999887, 9.124999997268817609, 0.000000000000000000 ) ) ;
#23050=CARTESIAN_POINT ( 'NONE',  ( 23.41746825000000243, 13.22499999726881192, -7.608796670333727974 ) ) ;
#23051=CARTESIAN_POINT ( 'NONE',  ( 18.94512977948575738, 6.424999997268809437, 13.76444248337723408 ) ) ;
#23064=CARTESIAN_POINT ( 'NONE',  ( 23.41746825000000243, 6.524999997268818852, 7.608796670333735079 ) ) ;
#23085=CARTESIAN_POINT ( 'NONE',  ( 24.50000000000000000, 15.74999999453763344, 0.000000000000000000 ) ) ;
#23101=CARTESIAN_POINT ( 'NONE',  ( 23.41746824999999887, 11.12499999726881938, 0.000000000000000000 ) ) ;
#23113=CARTESIAN_POINT ( 'NONE',  ( -4.223320258572819786E-15, 11.24999999453762456, 24.50000000000000000 ) ) ;
#23132=CARTESIAN_POINT ( 'NONE',  ( -23.41746824999999887, 15.52499999726882507, -7.608796670333730638 ) ) ;
#23139=CARTESIAN_POINT ( 'NONE',  ( 3.000384657911015469E-15, 16.99999999999998579, 24.50000000000000000 ) ) ;
#23152=VERTEX_POINT ( 'NONE', #15592 ) ;
#23172=CARTESIAN_POINT ( 'NONE',  ( -15.14183272437242600, 1.299999999999988054, 20.84094480462497856 ) ) ;
#23197=CARTESIAN_POINT ( 'NONE',  ( 14.47279130897151944, 9.424999997268814766, -19.92008829642072598 ) ) ;
#23227=CARTESIAN_POINT ( 'NONE',  ( 23.41746825000000243, 13.02499999726881619, 7.608796670333735079 ) ) ;
#23228=CARTESIAN_POINT ( 'NONE',  ( 18.94512977948575738, 2.424999997268806329, 13.76444248337723408 ) ) ;
#23242=CARTESIAN_POINT ( 'NONE',  ( -7.236395654485763274, 12.02499999726880375, 22.27133577429736633 ) ) ;
#23266=CARTESIAN_POINT ( 'NONE',  ( -24.50000000000000355, 10.64999999453762491, -7.960532557706207157 ) ) ;
#23273=CARTESIAN_POINT ( 'NONE',  ( -19.82091636218621034, 6.800000000000000711, -14.40073868116559552 ) ) ;
#23279=CARTESIAN_POINT ( 'NONE',  ( -23.41746824999999887, 6.124999997268814944, -2.867812753649727150E-15 ) ) ;
#23289=CARTESIAN_POINT ( 'NONE',  ( 19.82091636218621034, 9.800000000000002487, 14.40073868116559730 ) ) ;
#23303=SHAPE_DEFINITION_REPRESENTATION ( #3342, #33740 ) ;
#23308=AXIS2_PLACEMENT_3D ( 'NONE', #13537, #24000, #18853 ) ;
#23320=CARTESIAN_POINT ( 'NONE',  ( 3.245314017740486554E-15, -22.99999999999999289, 26.50000000000000355 ) ) ;
#23321=CARTESIAN_POINT ( 'NONE',  ( -24.50000000000000711, 12.84999999453761532, 7.960532557706201828 ) ) ;
#23333=ORIENTED_EDGE ( 'NONE', *, *, #24981, .T. ) ;
#23336=ORIENTED_EDGE ( 'NONE', *, *, #10326, .F. ) ;
#23342=AXIS2_PLACEMENT_3D ( 'NONE', #30064, #1575, #3826 ) ;
#23350=CARTESIAN_POINT ( 'NONE',  ( 19.82091636218621034, 7.800000000000001599, 14.40073868116559730 ) ) ;
#23355=CARTESIAN_POINT ( 'NONE',  ( 0.000000000000000000, 16.99999999999998579, 0.000000000000000000 ) ) ;
#23372=CARTESIAN_POINT ( 'NONE',  ( -18.94512977948575738, 9.924999997268812990, -13.76444248337723231 ) ) ;
#23373=VERTEX_POINT ( 'NONE', #1110 ) ;
#23389=CARTESIAN_POINT ( 'NONE',  ( 7.236395654485755280, 4.224999997268802154, 22.27133577429736988 ) ) ;
#23399=CARTESIAN_POINT ( 'NONE',  ( 18.94512977948575738, 14.92499999726881654, 13.76444248337723408 ) ) ;
#23400=CARTESIAN_POINT ( 'NONE',  ( 14.47279130897151767, 6.324999997268824892, 19.92008829642072953 ) ) ;
#23411=CARTESIAN_POINT ( 'NONE',  ( -7.236395654485763274, 8.024999997268828622, 22.27133577429736633 ) ) ;
#23419=VECTOR ( 'NONE', #6463, 1000.000000000000000 ) ;
#23427=CARTESIAN_POINT ( 'NONE',  ( -24.50000000000000000, 6.649999994537635573, -7.960532557706207157 ) ) ;
#23432=CARTESIAN_POINT ( 'NONE',  ( -24.50000000000000000, 15.00000000000001421, -3.000384657911015469E-15 ) ) ;
#23437=CARTESIAN_POINT ( 'NONE',  ( -15.14183272437241889, 10.44999999453763095, -20.84094480462497856 ) ) ;
#23452=CARTESIAN_POINT ( 'NONE',  ( -18.94512977948575738, 9.924999997268812990, -13.76444248337723231 ) ) ;
#23459=EDGE_LOOP ( 'NONE', ( #1993, #30715, #4880, #21058 ) ) ;
#23486=CARTESIAN_POINT ( 'NONE',  ( 1.415442245121193876, 16.99999999999998934, -23.63911378103994920 ) ) ;
#23500=ORIENTED_EDGE ( 'NONE', *, *, #23857, .F. ) ;
#23516=CARTESIAN_POINT ( 'NONE',  ( -7.570916362186210335, 2.599999999999991207, -23.30088464923126779 ) ) ;
#23517=( BOUNDED_CURVE ( )  B_SPLINE_CURVE ( 2, ( #1753, #14986, #25456, #1932, #18083, #3255, #10186, #31897, #4684, #31109, #327, #30937, #9834, #29155, #10015, #15511, #10980, #20669, #23228, #5026, #18719, #3094, #7430, #2457, #17917, #7603, #20311, #10814, #25792, #20486, #5661, #28369, #15163, #28531, #25629, #4857, #30761, #21294, #2108, #17738, #31734, #12581, #2281, #25963, #15337, #16144, #13565, #26597, #33687, #24028, #497, #7251, #21454, #28196, #12923, #12756, #8393, #23400, #23051, #8225, #18878, #29327, #5829, #16308, #26763, #13725, #24190, #33510, #11639, #8728, #6498, #11812, #24849, #6661, #27092, #8895, #14058, #14562, #32733, #19546, #3586, #22288, #14393, #11310, #29825, #32064, #16806, #19212, #11475, #29649, #6329, #24520, #9065, #19379, #990, #5990, #32566, #26922, #3418, #27262, #662, #3753, #29487, #11150, #6152, #21621, #14227, #24683, #27596, #21949, #9226, #16467, #32400, #1157, #21788, #8564, #29994, #829, #22123, #1329, #16971, #16636, #19048, #27429, #19710, #3920, #30156, #32236, #17143, #4087, #13892, #24359, #28111, #33598, #15075, #17650, #10098, #6825, #6999, #27943, #2021, #20398, #1669, #4939, #25543, #4256, #22793, #30849, #12496, #23132, #9921, #17481, #12663, #18003, #2189, #9744, #33424, #7168, #33246, #30329, #1501, #20230, #4426, #7340, #30670 ),
 .UNSPECIFIED., .F., .F. ) 
 B_SPLINE_CURVE_WITH_KNOTS ( ( 3, 2, 2, 2, 2, 2, 2, 2, 2, 2, 2, 2, 2, 2, 2, 2, 2, 2, 2, 2, 2, 2, 2, 2, 2, 2, 2, 2, 2, 2, 2, 2, 2, 2, 2, 2, 2, 2, 2, 2, 2, 2, 2, 2, 2, 2, 2, 2, 2, 2, 2, 2, 2, 2, 2, 2, 2, 2, 2, 2, 2, 2, 2, 2, 2, 2, 2, 2, 2, 2, 2, 2, 2, 2, 2, 2, 2, 2, 2, 2, 2, 2, 3 ),
 ( 0.000000000000000000, 0.01111111111111111154, 0.02222222222222222307, 0.03333333333333333287, 0.04444444444444444614, 0.05555555555555555247, 0.06666666666666666574, 0.07777777777777777901, 0.08888888888888889228, 0.1000000000000000056, 0.1111111111111111049, 0.1222222222222222182, 0.1333333333333333315, 0.1444444444444444309, 0.1555555555555555580, 0.1666666666666666574, 0.1777777777777777846, 0.1888888888888888840, 0.2000000000000000111, 0.2111111111111111105, 0.2222222222222222099, 0.2333333333333333370, 0.2444444444444444364, 0.2555555555555555358, 0.2666666666666666630, 0.2777777777777777901, 0.2888888888888888618, 0.2999999999999999889, 0.3111111111111111160, 0.3222222222222222432, 0.3333333333333333148, 0.3444444444444444420, 0.3555555555555555691, 0.3666666666666666408, 0.3777777777777777679, 0.3888888888888888951, 0.4000000000000000222, 0.4111111111111110938, 0.4222222222222222210, 0.4333333333333334036, 0.4444444444444444198, 0.4555555555555555469, 0.4666666666666666741, 0.4777777777777777457, 0.4888888888888888729, 0.5000000000000000000, 0.5111111111111110716, 0.5222222222222222543, 0.5333333333333333259, 0.5444444444444443976, 0.5555555555555555802, 0.5666666666666666519, 0.5777777777777777235, 0.5888888888888889062, 0.5999999999999999778, 0.6111111111111111605, 0.6222222222222222321, 0.6333333333333331927, 0.6444444444444444864, 0.6555555555555555580, 0.6666666666666666297, 0.6777777777777778123, 0.6888888888888888840, 0.6999999999999999556, 0.7111111111111111382, 0.7222222222222222099, 0.7333333333333332815, 0.7444444444444444642, 0.7555555555555555358, 0.7666666666666667185, 0.7777777777777777901, 0.7888888888888888618, 0.8000000000000000444, 0.8111111111111111160, 0.8222222222222221877, 0.8333333333333333703, 0.8444444444444444420, 0.8555555555555555136, 0.8666666666666668073, 0.8777777777777777679, 0.8888888888888888395, 0.9000000000000000222, 0.9096763566646446364 ),
 .UNSPECIFIED. ) 
 CURVE ( )  GEOMETRIC_REPRESENTATION_ITEM ( )  RATIONAL_B_SPLINE_CURVE ( ( 1.000000000000000000, 0.9510565162951535312, 1.000000000000000000, 0.9510565162951535312, 1.000000000000000000, 0.9510565162951535312, 1.000000000000000000, 0.9510565162951535312, 1.000000000000000000, 0.9510565162951535312, 1.000000000000000000, 0.9510565162951535312, 1.000000000000000000, 0.9510565162951535312, 1.000000000000000000, 0.9510565162951535312, 1.000000000000000000, 0.9510565162951535312, 1.000000000000000000, 0.9510565162951535312, 1.000000000000000000, 0.9510565162951535312, 1.000000000000000000, 0.9510565162951535312, 1.000000000000000000, 0.9510565162951535312, 1.000000000000000000, 0.9510565162951535312, 1.000000000000000000, 0.9510565162951535312, 1.000000000000000000, 0.9510565162951535312, 1.000000000000000000, 0.9510565162951535312, 1.000000000000000000, 0.9510565162951535312, 1.000000000000000000, 0.9510565162951535312, 1.000000000000000000, 0.9510565162951535312, 1.000000000000000000, 0.9510565162951535312, 1.000000000000000000, 0.9510565162951535312, 1.000000000000000000, 0.9510565162951535312, 1.000000000000000000, 0.9510565162951535312, 1.000000000000000000, 0.9510565162951535312, 1.000000000000000000, 0.9510565162951535312, 1.000000000000000000, 0.9510565162951535312, 1.000000000000000000, 0.9510565162951535312, 1.000000000000000000, 0.9510565162951535312, 1.000000000000000000, 0.9510565162951535312, 1.000000000000000000, 0.9510565162951535312, 1.000000000000000000, 0.9510565162951535312, 1.000000000000000000, 0.9510565162951535312, 1.000000000000000000, 0.9510565162951535312, 1.000000000000000000, 0.9510565162951535312, 1.000000000000000000, 0.9510565162951535312, 1.000000000000000000, 0.9510565162951535312, 1.000000000000000000, 0.9510565162951535312, 1.000000000000000000, 0.9510565162951535312, 1.000000000000000000, 0.9510565162951535312, 1.000000000000000000, 0.9510565162951535312, 1.000000000000000000, 0.9510565162951535312, 1.000000000000000000, 0.9510565162951535312, 1.000000000000000000, 0.9510565162951535312, 1.000000000000000000, 0.9510565162951535312, 1.000000000000000000, 0.9510565162951535312, 1.000000000000000000, 0.9510565162951535312, 1.000000000000000000, 0.9510565162951535312, 1.000000000000000000, 0.9510565162951535312, 1.000000000000000000, 0.9510565162951535312, 1.000000000000000000, 0.9510565162951535312, 1.000000000000000000, 0.9510565162951535312, 1.000000000000000000, 0.9510565162951535312, 1.000000000000000000, 0.9510565162951535312, 1.000000000000000000, 0.9510565162951535312, 1.000000000000000000, 0.9510565162951535312, 1.000000000000000000, 0.9510565162951535312, 1.000000000000000000, 0.9510565162951535312, 1.000000000000000000, 0.9510565162951535312, 1.000000000000000000, 0.9510565162951535312, 1.000000000000000000, 0.9510565162951535312, 1.000000000000000000, 0.9510565162951535312, 1.000000000000000000, 0.9510565162951535312, 1.000000000000000000, 0.9510565162951535312, 1.000000000000000000, 0.9510565162951535312, 1.000000000000000000, 0.9510565162951535312, 1.000000000000000000, 0.9510565162951535312, 1.000000000000000000, 0.9510565162951535312, 1.000000000000000000, 0.9510565162951535312, 1.000000000000000000, 0.9510565162951535312, 1.000000000000000000, 0.9510565162951535312, 1.000000000000000000, 0.9510565162951535312, 1.000000000000000000, 0.9510565162951535312, 1.000000000000000000, 0.9510565162951535312, 1.000000000000000000, 0.9510565162951535312, 1.000000000000000000, 0.9510565162951535312, 1.000000000000000000, 0.9510565162951535312, 1.000000000000000000, 0.9510565162951535312, 1.000000000000000000, 0.9510565162951535312, 1.000000000000000000, 0.9510565162951535312, 1.000000000000000000, 0.9510565162951535312, 1.000000000000000000, 0.9573764855735513724, 0.9889922301674725080 ) ) 
 REPRESENTATION_ITEM ( '' )  );
#23519=CARTESIAN_POINT ( 'NONE',  ( 7.570916362186213000, 2.149999994537632464, -23.30088464923126423 ) ) ;
#23522=DIRECTION ( 'NONE',  ( 0.000000000000000000, 0.000000000000000000, -1.000000000000000000 ) ) ;
#23542=CARTESIAN_POINT ( 'NONE',  ( -23.41746824999999887, 12.02499999726881974, -7.608796670333730638 ) ) ;
#23558=CARTESIAN_POINT ( 'NONE',  ( 14.47279130897151589, 6.324999997268824892, 19.92008829642072953 ) ) ;
#23567=CARTESIAN_POINT ( 'NONE',  ( -14.47279130897152122, 18.42499999726882365, 19.92008829642072243 ) ) ;
#23579=CARTESIAN_POINT ( 'NONE',  ( 14.47279130897151767, 8.924999997268800556, -19.92008829642072598 ) ) ;
#23594=CARTESIAN_POINT ( 'NONE',  ( -7.570916362186210335, 6.349999994537613546, -23.30088464923126779 ) ) ;
#23603=CARTESIAN_POINT ( 'NONE',  ( 15.14183272437242245, 14.04999999453763593, -20.84094480462497856 ) ) ;
#23617=CARTESIAN_POINT ( 'NONE',  ( 23.41746825000000243, 9.224999997268820806, -7.608796670333727974 ) ) ;
#23683=CARTESIAN_POINT ( 'NONE',  ( 19.82091636218621389, 8.200000000000013500, -14.40073868116559197 ) ) ;
#23692=CARTESIAN_POINT ( 'NONE',  ( 15.14183272437242067, 9.449999994537636283, 20.84094480462498211 ) ) ;
#23707=CARTESIAN_POINT ( 'NONE',  ( 14.47279130897151944, 13.42499999726880411, -19.92008829642072598 ) ) ;
#23724=CARTESIAN_POINT ( 'NONE',  ( 14.47279130897151767, 4.924999997268811214, -19.92008829642072598 ) ) ;
#23748=CARTESIAN_POINT ( 'NONE',  ( -14.47279130897152122, 11.92499999726882010, 19.92008829642072243 ) ) ;
#23769=CARTESIAN_POINT ( 'NONE',  ( -3.880418787951104953, 15.44874571845315359, 24.50000000000000711 ) ) ;
#23776=CARTESIAN_POINT ( 'NONE',  ( -7.236395654485763274, 2.524999997268823293, 22.27133577429736633 ) ) ;
#23791=CARTESIAN_POINT ( 'NONE',  ( -4.523095164977116484E-15, 10.62499999726880695, 24.62258325217400312 ) ) ;
#23841=ORIENTED_EDGE ( 'NONE', *, *, #12073, .F. ) ;
#23846=LINE ( 'NONE', #29311, #28896 ) ;
#23856=CARTESIAN_POINT ( 'NONE',  ( 15.14183272437242245, 4.300000000000009592, -20.84094480462497856 ) ) ;
#23857=EDGE_CURVE ( 'NONE', #10883, #14840, #23517, .T. ) ;
#23859=CARTESIAN_POINT ( 'NONE',  ( 7.570916362186207671, 3.349999994537639303, 23.30088464923126779 ) ) ;
#23862=FACE_OUTER_BOUND ( 'NONE', #27330, .T. ) ;
#23878=CARTESIAN_POINT ( 'NONE',  ( 14.47279130897151944, 11.42499999726880944, -19.92008829642072598 ) ) ;
#23888=LINE ( 'NONE', #20816, #13231 ) ;
#23894=CARTESIAN_POINT ( 'NONE',  ( -23.41746825000000243, 5.524999997268821517, -7.608796670333730638 ) ) ;
#23903=CARTESIAN_POINT ( 'NONE',  ( -18.94512977948576093, 18.32499999726880446, 13.76444248337722698 ) ) ;
#23925=ADVANCED_FACE ( 'NONE', ( #1844 ), #28282, .T. ) ;
#23944=CARTESIAN_POINT ( 'NONE',  ( 19.82091636218621034, 19.54999999453763238, 14.40073868116559730 ) ) ;
#23957=CARTESIAN_POINT ( 'NONE',  ( -23.41746825000000598, 16.22499999726880304, 7.608796670333726198 ) ) ;
#24000=DIRECTION ( 'NONE',  ( -0.000000000000000000, 1.000000000000000000, -0.000000000000000000 ) ) ;
#24022=CARTESIAN_POINT ( 'NONE',  ( 15.14183272437241889, 3.699999999999999289, 20.84094480462498211 ) ) ;
#24028=CARTESIAN_POINT ( 'NONE',  ( -23.41746824999999887, 5.524999997268821517, -7.608796670333730638 ) ) ;
#24029=CARTESIAN_POINT ( 'NONE',  ( -15.14183272437242067, 8.700000000000017053, -20.84094480462497856 ) ) ;
#24046=CARTESIAN_POINT ( 'NONE',  ( 18.94512977948575738, 14.92499999726881654, 13.76444248337723408 ) ) ;
#24060=EDGE_CURVE ( 'NONE', #28296, #21102, #25365, .T. ) ;
#24065=CARTESIAN_POINT ( 'NONE',  ( 23.41746825000000243, 6.724999997268811924, -7.608796670333727974 ) ) ;
#24086=CARTESIAN_POINT ( 'NONE',  ( 23.41746825000000243, 12.52499999726880375, 7.608796670333735079 ) ) ;
#24093=VERTEX_POINT ( 'NONE', #15421 ) ;
#24110=CARTESIAN_POINT ( 'NONE',  ( 24.50000000000000000, 17.74999999453763522, 0.000000000000000000 ) ) ;
#24125=CARTESIAN_POINT ( 'NONE',  ( 23.41746824999999887, 15.12499999726882294, 0.000000000000000000 ) ) ;
#24126=VERTEX_POINT ( 'NONE', #115 ) ;
#24133=CARTESIAN_POINT ( 'NONE',  ( -6.668400408272875007E-16, 0.5000000000000068834, -24.50000000000000355 ) ) ;
#24148=CARTESIAN_POINT ( 'NONE',  ( -24.50000000000000000, 11.00000000000001066, -3.000384657911015469E-15 ) ) ;
#24158=CARTESIAN_POINT ( 'NONE',  ( 15.14183272437242067, 11.44999999453763095, 20.84094480462498211 ) ) ;
#24170=EDGE_LOOP ( 'NONE', ( #32795, #14290, #17541, #3336 ) ) ;
#24186=CARTESIAN_POINT ( 'NONE',  ( -24.50000000000000000, 13.00000000000001066, -3.000384657911015469E-15 ) ) ;
#24188=CARTESIAN_POINT ( 'NONE',  ( -24.50000000000001066, 6.849999994537628645, 7.960532557706201828 ) ) ;
#24190=CARTESIAN_POINT ( 'NONE',  ( -7.236395654485757944, 7.224999997268804819, -22.27133577429736988 ) ) ;
#24196=CARTESIAN_POINT ( 'NONE',  ( 23.22858344560803445, 16.99999999999999289, -3.065087378623344794 ) ) ;
#24227=CARTESIAN_POINT ( 'NONE',  ( -14.47279130897151589, 13.32499999726880624, -19.92008829642072598 ) ) ;
#24234=ORIENTED_EDGE ( 'NONE', *, *, #4893, .F. ) ;
#24235=DIRECTION ( 'NONE',  ( 0.000000000000000000, 0.000000000000000000, -1.000000000000000000 ) ) ;
#24248=CARTESIAN_POINT ( 'NONE',  ( -23.41746825000000243, 13.52499999726880198, -7.608796670333730638 ) ) ;
#24276=CARTESIAN_POINT ( 'NONE',  ( -7.236395654485757944, 1.724999997268800156, -22.27133577429736988 ) ) ;
#24293=CARTESIAN_POINT ( 'NONE',  ( -23.41746825000000243, 14.02499999726881263, -7.608796670333730638 ) ) ;
#24322=CARTESIAN_POINT ( 'NONE',  ( 7.736786493336079928, 16.99999999999999645, 22.60298709876044398 ) ) ;
#24343=CARTESIAN_POINT ( 'NONE',  ( 19.82091636218621034, 15.54999999453762705, 14.40073868116559730 ) ) ;
#24344=EDGE_CURVE ( 'NONE', #16549, #2430, #32816, .T. ) ;
#24356=CARTESIAN_POINT ( 'NONE',  ( -19.82091636218621389, 13.19999999999998863, 14.40073868116558842 ) ) ;
#24359=CARTESIAN_POINT ( 'NONE',  ( -23.41746825000000243, 13.72499999726882258, 7.608796670333725309 ) ) ;
#24372=CARTESIAN_POINT ( 'NONE',  ( -15.14183272437242067, 16.69999999999999574, -20.84094480462497856 ) ) ;
#24377=CYLINDRICAL_SURFACE ( 'NONE', #10271, 26.50000000000000355 ) ;
#24389=CARTESIAN_POINT ( 'NONE',  ( -14.47279130897151589, 11.32499999726881157, -19.92008829642072598 ) ) ;
#24409=CARTESIAN_POINT ( 'NONE',  ( 23.41746824999999887, 14.62499999726882294, 0.000000000000000000 ) ) ;
#24424=DIRECTION ( 'NONE',  ( -0.000000000000000000, -1.000000000000000000, -0.000000000000000000 ) ) ;
#24434=CARTESIAN_POINT ( 'NONE',  ( -7.236395654485763274, 6.524999997268826846, 22.27133577429736633 ) ) ;
#24450=CARTESIAN_POINT ( 'NONE',  ( -23.41746825000000598, 14.22499999726880660, 7.608796670333726198 ) ) ;
#24466=ADVANCED_FACE ( 'NONE', ( #32693 ), #11278, .T. ) ;
#24492=CARTESIAN_POINT ( 'NONE',  ( -15.14183272437242778, 13.29999999999998650, 20.84094480462497856 ) ) ;
#24516=CARTESIAN_POINT ( 'NONE',  ( -15.14183272437241889, 14.70000000000000107, -20.84094480462497856 ) ) ;
#24520=CARTESIAN_POINT ( 'NONE',  ( -23.41746825000000243, 9.724999997268803043, 7.608796670333725309 ) ) ;
#24521=CARTESIAN_POINT ( 'NONE',  ( 3.880418787951134707, 3.551254281546844194, 24.50000000000000000 ) ) ;
#24537=DIRECTION ( 'NONE',  ( 0.000000000000000000, -1.000000000000000000, 0.000000000000000000 ) ) ;
#24551=CARTESIAN_POINT ( 'NONE',  ( 14.47279130897151589, 12.32499999726880802, 19.92008829642072953 ) ) ;
#24573=CARTESIAN_POINT ( 'NONE',  ( -23.41746825000000598, 17.72499999726881725, 7.608796670333726198 ) ) ;
#24577=CARTESIAN_POINT ( 'NONE',  ( -23.41746824999999887, 4.024999997268810858, -7.608796670333730638 ) ) ;
#24588=CARTESIAN_POINT ( 'NONE',  ( 0.000000000000000000, 16.99999999999998579, 0.000000000000000000 ) ) ;
#24598=CARTESIAN_POINT ( 'NONE',  ( 23.41746825000000243, 7.024999997268802865, 7.608796670333735079 ) ) ;
#24613=CARTESIAN_POINT ( 'NONE',  ( -4.523095164977116484E-15, 16.62499999726881583, 24.62258325217400312 ) ) ;
#24642=CARTESIAN_POINT ( 'NONE',  ( -10.86059781102998478, 16.99999999999999289, 21.84823680246600119 ) ) ;
#24644=CARTESIAN_POINT ( 'NONE',  ( 24.50000000000000000, 11.64999999453762314, 7.960532557706212486 ) ) ;
#24679=CARTESIAN_POINT ( 'NONE',  ( 24.50000000000000000, 14.00000000000001243, 0.000000000000000000 ) ) ;
#24683=CARTESIAN_POINT ( 'NONE',  ( -14.47279130897151767, 11.32499999726881157, -19.92008829642072598 ) ) ;
#24684=CARTESIAN_POINT ( 'NONE',  ( -24.50000000000000000, 9.000000000000007105, -3.000384657911015469E-15 ) ) ;
#24716=CARTESIAN_POINT ( 'NONE',  ( 14.47279130897151589, 8.324999997268818674, 19.92008829642072953 ) ) ;
#24719=VECTOR ( 'NONE', #15095, 1000.000000000000000 ) ;
#24741=CARTESIAN_POINT ( 'NONE',  ( 23.41746824999999887, 3.224999997268806151, -7.608796670333727974 ) ) ;
#24746=EDGE_CURVE ( 'NONE', #3731, #5367, #17608, .T. ) ;
#24753=DIRECTION ( 'NONE',  ( 0.000000000000000000, 0.000000000000000000, -1.000000000000000000 ) ) ;
#24763=CARTESIAN_POINT ( 'NONE',  ( 18.94512977948575738, 6.924999997268810326, 13.76444248337723408 ) ) ;
#24777=CARTESIAN_POINT ( 'NONE',  ( 23.41746825000000243, 2.724999997268822138, -7.608796670333727974 ) ) ;
#24787=VERTEX_POINT ( 'NONE', #26009 ) ;
#24795=EDGE_CURVE ( 'NONE', #21231, #31792, #10891, .T. ) ;
#24803=CARTESIAN_POINT ( 'NONE',  ( 7.570916362186207671, 9.349999994537617098, 23.30088464923126779 ) ) ;
#24811=CARTESIAN_POINT ( 'NONE',  ( 3.503834181885622456, 16.99999999999998934, 23.74784554439683149 ) ) ;
#24845=CARTESIAN_POINT ( 'NONE',  ( 24.50000000000000355, 9.900000000000007461, 7.960532557706212486 ) ) ;
#24849=CARTESIAN_POINT ( 'NONE',  ( -18.94512977948576093, 7.824999997268822227, 13.76444248337722698 ) ) ;
#24853=CARTESIAN_POINT ( 'NONE',  ( -24.50000000000000000, 4.649999994537640902, -7.960532557706207157 ) ) ;
#24868=ORIENTED_EDGE ( 'NONE', *, *, #31186, .T. ) ;
#24883=CARTESIAN_POINT ( 'NONE',  ( -18.94512977948576093, 11.82499999726882578, 13.76444248337722698 ) ) ;
#24889=VERTEX_POINT ( 'NONE', #21044 ) ;
#24931=CARTESIAN_POINT ( 'NONE',  ( -14.47279130897152122, 8.424999997268816543, 19.92008829642072243 ) ) ;
#24947=CARTESIAN_POINT ( 'NONE',  ( 1.507698388325705758E-15, 1.124999997268814722, -24.62258325217400312 ) ) ;
#24959=( GEOMETRIC_REPRESENTATION_CONTEXT ( 3 ) GLOBAL_UNCERTAINTY_ASSIGNED_CONTEXT ( ( #33516 ) ) GLOBAL_UNIT_ASSIGNED_CONTEXT ( ( #16877, #3495, #27676 ) ) REPRESENTATION_CONTEXT ( 'NONE', 'WORKASPACE' ) );
#24972=CARTESIAN_POINT ( 'NONE',  ( 24.50000000000000000, 3.749999994537622783, 0.000000000000000000 ) ) ;
#24981=EDGE_CURVE ( 'NONE', #24889, #27958, #17919, .T. ) ;
#24988=CARTESIAN_POINT ( 'NONE',  ( -23.41746825000000243, 2.024999997268815299, -7.608796670333730638 ) ) ;
#25001=CARTESIAN_POINT ( 'NONE',  ( -24.50000000000000000, 8.749999994537628112, -3.000384657911015469E-15 ) ) ;
#25025=CARTESIAN_POINT ( 'NONE',  ( 21.64573397815488676, 16.99999999999998579, 8.935324268693841887 ) ) ;
#25040=CARTESIAN_POINT ( 'NONE',  ( 0.000000000000000000, -20.99999999999998934, 0.000000000000000000 ) ) ;
#25055=CARTESIAN_POINT ( 'NONE',  ( 15.14183272437241889, 1.700000000000004396, 20.84094480462498211 ) ) ;
#25077=CARTESIAN_POINT ( 'NONE',  ( -23.41746824999999887, 2.124999997268811391, -2.867812753649727150E-15 ) ) ;
#25103=( BOUNDED_SURFACE ( )  B_SPLINE_SURFACE ( 1, 2, ( 
 ( #15801, #7722, #13209, #13047, #23519, #28484, #10640, #33978, #20950, #31562, #31399, #7889, #26257, #5490, #15969, #13386, #23859, #4378, #14853, #14513, #24972, #25319, #12271, #33019, #1620, #32850, #3253, #29324, #1454, #27551, #22745, #19665, #6950, #13723, #6614, #9345, #6452, #18875, #4211, #19500, #11933, #20006, #30110, #22241, #33196, #9525, #30453, #30280, #5826, #4039, #17434, #24188, #27895, #27723, #29948, #1793, #9181, #14683, #16926, #27384, #3873, #22402, #17092, #19828, #6782, #16305, #17260, #660, #9018, #26761, #25144, #11148, #22074, #12098, #32519, #14347, #24803, #22569, #1281, #11760, #32686, #28741, #5237, #4894, #15374, #15721, #2670, #23437, #26001, #23266, #28063, #28404, #12792, #33728, #20348, #7473, #10226, #30973, #7119, #7807, #7639, #12449, #17955, #26176, #10389, #15200, #4550, #13129, #22919, #20706, #33548, #25829, #20530, #2319, #31148, #15029, #25494, #18123, #17601, #28568, #33375, #5064, #15549, #23603, #2494, #9870, #12963, #33898, #20867, #31315, #10049, #30798, #18296, #9699, #20179, #30623, #25664, #1974, #2143, #7291, #23085, #17776, #28234, #4720, #12618, #18966, #21037, #5746, #29410, #13971, #3007, #3177, #28907, #70, #18636, #13808, #16389, #13646, #18463, #18798, #24110, #578, #10728, #31816, #11068, #21372, #31487, #32151, #31982, #2832, #8307, #16550, #744, #5577, #5408, #19129, #13301, #21534, #23944, #16227, #10899 ),
 ( #29073, #15887, #13479, #8479, #29566, #26343, #24276, #7977, #26681, #6067, #26513, #5912, #413, #10558, #23776, #26842, #242, #3337, #21205, #31649, #8147, #11229, #21705, #29242, #27003, #8644, #16058, #3501, #19967, #27175, #14647, #1241, #1582, #9305, #17224, #14142, #19789, #27858, #3833, #27513, #27683, #16884, #4173, #32317, #14474, #4340, #29909, #6239, #11390, #14307, #30413, #32980, #19291, #32812, #24434, #4001, #19461, #27347, #24763, #24598, #21867, #9484, #6913, #25106, #8808, #17394, #8979, #1072, #22202, #6577, #17051, #6412, #11552, #24931, #11719, #30238, #12059, #16720, #22365, #1416, #32649, #22529, #3668, #6743, #911, #29734, #22034, #32478, #11894, #9143, #19626, #30071, #25628, #28368, #30586, #10014, #12409, #25791, #4511, #17916, #2280, #10354, #12755, #14985, #20668, #31108, #7602, #4856, #15162, #25455, #18082, #2456, #28703, #30936, #20310, #20485, #30760, #12922, #28195, #23227, #1752, #23050, #12580, #33686, #12232, #7429, #10185, #14814, #17737, #15336, #9661, #25279, #33336, #22706, #28530, #33509, #7770, #2107, #23399, #20142, #5025, #15510, #1931, #33158, #25962, #22879, #33860, #20832, #31277, #4683, #7082, #18257, #17566, #28023, #9833, #7250, #5871, #10521, #29372, #13608, #15849, #21662, #29035, #539, #26305, #5368, #2794, #8268, #26473, #2967, #13436, #15684, #23903, #23567, #28872, #32107, #375, #3300, #26134, #10860, #18925 ) ),
 .UNSPECIFIED., .F., .F., .T. ) 
 B_SPLINE_SURFACE_WITH_KNOTS ( ( 2, 2 ),
 ( 3, 2, 2, 2, 2, 2, 2, 2, 2, 2, 2, 2, 2, 2, 2, 2, 2, 2, 2, 2, 2, 2, 2, 2, 2, 2, 2, 2, 2, 2, 2, 2, 2, 2, 2, 2, 2, 2, 2, 2, 2, 2, 2, 2, 2, 2, 2, 2, 2, 2, 2, 2, 2, 2, 2, 2, 2, 2, 2, 2, 2, 2, 2, 2, 2, 2, 2, 2, 2, 2, 2, 2, 2, 2, 2, 2, 2, 2, 2, 2, 2, 2, 2, 2, 2, 2, 2, 2, 2, 2, 3 ),
 ( 0.000000000000000000, 1.000000000000000000 ),
 ( 0.000000000000000000, 0.01111111111111111154, 0.02222222222222222307, 0.03333333333333333287, 0.04444444444444444614, 0.05555555555555555247, 0.06666666666666666574, 0.07777777777777777901, 0.08888888888888889228, 0.1000000000000000056, 0.1111111111111111049, 0.1222222222222222182, 0.1333333333333333315, 0.1444444444444444309, 0.1555555555555555580, 0.1666666666666666574, 0.1777777777777777846, 0.1888888888888888840, 0.2000000000000000111, 0.2111111111111111105, 0.2222222222222222099, 0.2333333333333333370, 0.2444444444444444364, 0.2555555555555555358, 0.2666666666666666630, 0.2777777777777777901, 0.2888888888888888618, 0.2999999999999999889, 0.3111111111111111160, 0.3222222222222222432, 0.3333333333333333148, 0.3444444444444444420, 0.3555555555555555691, 0.3666666666666666408, 0.3777777777777777679, 0.3888888888888888951, 0.4000000000000000222, 0.4111111111111110938, 0.4222222222222222210, 0.4333333333333333481, 0.4444444444444444198, 0.4555555555555555469, 0.4666666666666666741, 0.4777777777777778012, 0.4888888888888888729, 0.5000000000000000000, 0.5111111111111110716, 0.5222222222222222543, 0.5333333333333333259, 0.5444444444444443976, 0.5555555555555555802, 0.5666666666666666519, 0.5777777777777777235, 0.5888888888888889062, 0.5999999999999999778, 0.6111111111111111605, 0.6222222222222222321, 0.6333333333333333037, 0.6444444444444444864, 0.6555555555555555580, 0.6666666666666666297, 0.6777777777777778123, 0.6888888888888888840, 0.6999999999999999556, 0.7111111111111111382, 0.7222222222222222099, 0.7333333333333332815, 0.7444444444444444642, 0.7555555555555555358, 0.7666666666666667185, 0.7777777777777777901, 0.7888888888888888618, 0.8000000000000000444, 0.8111111111111111160, 0.8222222222222221877, 0.8333333333333333703, 0.8444444444444444420, 0.8555555555555555136, 0.8666666666666666963, 0.8777777777777777679, 0.8888888888888888395, 0.9000000000000000222, 0.9111111111111110938, 0.9222222222222222765, 0.9333333333333333481, 0.9444444444444444198, 0.9555555555555556024, 0.9666666666666666741, 0.9777777777777777457, 0.9888888888888889284, 1.000000000000000000 ),
 .UNSPECIFIED. ) 
 GEOMETRIC_REPRESENTATION_ITEM ( )  RATIONAL_B_SPLINE_SURFACE ( (
 ( 1.000000000000000000, 0.9510565162951535312, 1.000000000000000000, 0.9510565162951535312, 1.000000000000000000, 0.9510565162951535312, 1.000000000000000000, 0.9510565162951535312, 1.000000000000000000, 0.9510565162951535312, 1.000000000000000000, 0.9510565162951535312, 1.000000000000000000, 0.9510565162951535312, 1.000000000000000000, 0.9510565162951535312, 1.000000000000000000, 0.9510565162951535312, 1.000000000000000000, 0.9510565162951535312, 1.000000000000000000, 0.9510565162951535312, 1.000000000000000000, 0.9510565162951535312, 1.000000000000000000, 0.9510565162951535312, 1.000000000000000000, 0.9510565162951535312, 1.000000000000000000, 0.9510565162951535312, 1.000000000000000000, 0.9510565162951535312, 1.000000000000000000, 0.9510565162951535312, 1.000000000000000000, 0.9510565162951535312, 1.000000000000000000, 0.9510565162951535312, 1.000000000000000000, 0.9510565162951535312, 1.000000000000000000, 0.9510565162951535312, 1.000000000000000000, 0.9510565162951535312, 1.000000000000000000, 0.9510565162951535312, 1.000000000000000000, 0.9510565162951535312, 1.000000000000000000, 0.9510565162951535312, 1.000000000000000000, 0.9510565162951535312, 1.000000000000000000, 0.9510565162951535312, 1.000000000000000000, 0.9510565162951535312, 1.000000000000000000, 0.9510565162951535312, 1.000000000000000000, 0.9510565162951535312, 1.000000000000000000, 0.9510565162951535312, 1.000000000000000000, 0.9510565162951535312, 1.000000000000000000, 0.9510565162951535312, 1.000000000000000000, 0.9510565162951535312, 1.000000000000000000, 0.9510565162951535312, 1.000000000000000000, 0.9510565162951535312, 1.000000000000000000, 0.9510565162951535312, 1.000000000000000000, 0.9510565162951535312, 1.000000000000000000, 0.9510565162951535312, 1.000000000000000000, 0.9510565162951535312, 1.000000000000000000, 0.9510565162951535312, 1.000000000000000000, 0.9510565162951535312, 1.000000000000000000, 0.9510565162951535312, 1.000000000000000000, 0.9510565162951535312, 1.000000000000000000, 0.9510565162951535312, 1.000000000000000000, 0.9510565162951535312, 1.000000000000000000, 0.9510565162951535312, 1.000000000000000000, 0.9510565162951535312, 1.000000000000000000, 0.9510565162951535312, 1.000000000000000000, 0.9510565162951535312, 1.000000000000000000, 0.9510565162951535312, 1.000000000000000000, 0.9510565162951535312, 1.000000000000000000, 0.9510565162951535312, 1.000000000000000000, 0.9510565162951535312, 1.000000000000000000, 0.9510565162951535312, 1.000000000000000000, 0.9510565162951535312, 1.000000000000000000, 0.9510565162951535312, 1.000000000000000000, 0.9510565162951535312, 1.000000000000000000, 0.9510565162951535312, 1.000000000000000000, 0.9510565162951535312, 1.000000000000000000, 0.9510565162951535312, 1.000000000000000000, 0.9510565162951535312, 1.000000000000000000, 0.9510565162951535312, 1.000000000000000000, 0.9510565162951535312, 1.000000000000000000, 0.9510565162951535312, 1.000000000000000000, 0.9510565162951535312, 1.000000000000000000, 0.9510565162951535312, 1.000000000000000000, 0.9510565162951535312, 1.000000000000000000, 0.9510565162951535312, 1.000000000000000000, 0.9510565162951535312, 1.000000000000000000, 0.9510565162951535312, 1.000000000000000000, 0.9510565162951535312, 1.000000000000000000, 0.9510565162951535312, 1.000000000000000000, 0.9510565162951535312, 1.000000000000000000, 0.9510565162951535312, 1.000000000000000000, 0.9510565162951535312, 1.000000000000000000, 0.9510565162951535312, 1.000000000000000000, 0.9510565162951535312, 1.000000000000000000, 0.9510565162951535312, 1.000000000000000000, 0.9510565162951535312, 1.000000000000000000, 0.9510565162951535312, 1.000000000000000000, 0.9510565162951535312, 1.000000000000000000, 0.9510565162951535312, 1.000000000000000000, 0.9510565162951535312, 1.000000000000000000, 0.9510565162951535312, 1.000000000000000000, 0.9510565162951535312, 1.000000000000000000, 0.9510565162951535312, 1.000000000000000000, 0.9510565162951535312, 1.000000000000000000, 0.9510565162951535312, 1.000000000000000000, 0.9510565162951535312, 1.000000000000000000),
 ( 1.000000000000000000, 0.9510565162951535312, 1.000000000000000000, 0.9510565162951535312, 1.000000000000000000, 0.9510565162951535312, 1.000000000000000000, 0.9510565162951535312, 1.000000000000000000, 0.9510565162951535312, 1.000000000000000000, 0.9510565162951535312, 1.000000000000000000, 0.9510565162951535312, 1.000000000000000000, 0.9510565162951535312, 1.000000000000000000, 0.9510565162951535312, 1.000000000000000000, 0.9510565162951535312, 1.000000000000000000, 0.9510565162951535312, 1.000000000000000000, 0.9510565162951535312, 1.000000000000000000, 0.9510565162951535312, 1.000000000000000000, 0.9510565162951535312, 1.000000000000000000, 0.9510565162951535312, 1.000000000000000000, 0.9510565162951535312, 1.000000000000000000, 0.9510565162951535312, 1.000000000000000000, 0.9510565162951535312, 1.000000000000000000, 0.9510565162951535312, 1.000000000000000000, 0.9510565162951535312, 1.000000000000000000, 0.9510565162951535312, 1.000000000000000000, 0.9510565162951535312, 1.000000000000000000, 0.9510565162951535312, 1.000000000000000000, 0.9510565162951535312, 1.000000000000000000, 0.9510565162951535312, 1.000000000000000000, 0.9510565162951535312, 1.000000000000000000, 0.9510565162951535312, 1.000000000000000000, 0.9510565162951535312, 1.000000000000000000, 0.9510565162951535312, 1.000000000000000000, 0.9510565162951535312, 1.000000000000000000, 0.9510565162951535312, 1.000000000000000000, 0.9510565162951535312, 1.000000000000000000, 0.9510565162951535312, 1.000000000000000000, 0.9510565162951535312, 1.000000000000000000, 0.9510565162951535312, 1.000000000000000000, 0.9510565162951535312, 1.000000000000000000, 0.9510565162951535312, 1.000000000000000000, 0.9510565162951535312, 1.000000000000000000, 0.9510565162951535312, 1.000000000000000000, 0.9510565162951535312, 1.000000000000000000, 0.9510565162951535312, 1.000000000000000000, 0.9510565162951535312, 1.000000000000000000, 0.9510565162951535312, 1.000000000000000000, 0.9510565162951535312, 1.000000000000000000, 0.9510565162951535312, 1.000000000000000000, 0.9510565162951535312, 1.000000000000000000, 0.9510565162951535312, 1.000000000000000000, 0.9510565162951535312, 1.000000000000000000, 0.9510565162951535312, 1.000000000000000000, 0.9510565162951535312, 1.000000000000000000, 0.9510565162951535312, 1.000000000000000000, 0.9510565162951535312, 1.000000000000000000, 0.9510565162951535312, 1.000000000000000000, 0.9510565162951535312, 1.000000000000000000, 0.9510565162951535312, 1.000000000000000000, 0.9510565162951535312, 1.000000000000000000, 0.9510565162951535312, 1.000000000000000000, 0.9510565162951535312, 1.000000000000000000, 0.9510565162951535312, 1.000000000000000000, 0.9510565162951535312, 1.000000000000000000, 0.9510565162951535312, 1.000000000000000000, 0.9510565162951535312, 1.000000000000000000, 0.9510565162951535312, 1.000000000000000000, 0.9510565162951535312, 1.000000000000000000, 0.9510565162951535312, 1.000000000000000000, 0.9510565162951535312, 1.000000000000000000, 0.9510565162951535312, 1.000000000000000000, 0.9510565162951535312, 1.000000000000000000, 0.9510565162951535312, 1.000000000000000000, 0.9510565162951535312, 1.000000000000000000, 0.9510565162951535312, 1.000000000000000000, 0.9510565162951535312, 1.000000000000000000, 0.9510565162951535312, 1.000000000000000000, 0.9510565162951535312, 1.000000000000000000, 0.9510565162951535312, 1.000000000000000000, 0.9510565162951535312, 1.000000000000000000, 0.9510565162951535312, 1.000000000000000000, 0.9510565162951535312, 1.000000000000000000, 0.9510565162951535312, 1.000000000000000000, 0.9510565162951535312, 1.000000000000000000, 0.9510565162951535312, 1.000000000000000000, 0.9510565162951535312, 1.000000000000000000, 0.9510565162951535312, 1.000000000000000000, 0.9510565162951535312, 1.000000000000000000, 0.9510565162951535312, 1.000000000000000000, 0.9510565162951535312, 1.000000000000000000, 0.9510565162951535312, 1.000000000000000000, 0.9510565162951535312, 1.000000000000000000, 0.9510565162951535312, 1.000000000000000000, 0.9510565162951535312, 1.000000000000000000) ) ) 
 REPRESENTATION_ITEM ( '' )  SURFACE ( )  );
#25106=CARTESIAN_POINT ( 'NONE',  ( 14.47279130897151767, 7.424999997268820096, -19.92008829642072598 ) ) ;
#25119=CARTESIAN_POINT ( 'NONE',  ( -14.47279130897152122, 1.924999997268818541, 19.92008829642072243 ) ) ;
#25144=CARTESIAN_POINT ( 'NONE',  ( -24.50000000000000000, 8.749999994537628112, -3.000384657911015469E-15 ) ) ;
#25157=CARTESIAN_POINT ( 'NONE',  ( 23.41746824999999887, 3.124999997268812280, 0.000000000000000000 ) ) ;
#25169=CARTESIAN_POINT ( 'NONE',  ( -7.570916362186210335, 8.349999994537615322, -23.30088464923126779 ) ) ;
#25187=CARTESIAN_POINT ( 'NONE',  ( 7.570916362186207671, 15.60000000000000320, 23.30088464923126779 ) ) ;
#25195=CARTESIAN_POINT ( 'NONE',  ( 22.19496127021523435, 16.99999999999998579, 7.506443533373466259 ) ) ;
#25225=PRESENTATION_STYLE_ASSIGNMENT (( #4630 ) ) ;
#25230=CARTESIAN_POINT ( 'NONE',  ( -23.41746824999999887, 17.62499999726882649, -2.867812753649727150E-15 ) ) ;
#25236=ORIENTED_EDGE ( 'NONE', *, *, #9886, .T. ) ;
#25253=CARTESIAN_POINT ( 'NONE',  ( 14.47279130897151767, 6.824999997268808904, 19.92008829642072953 ) ) ;
#25254=ORIENTED_EDGE ( 'NONE', *, *, #2863, .F. ) ;
#25275=CARTESIAN_POINT ( 'NONE',  ( 24.50000000000000000, 8.000000000000007105, 0.000000000000000000 ) ) ;
#25279=CARTESIAN_POINT ( 'NONE',  ( -23.41746825000000598, 14.22499999726880660, 7.608796670333726198 ) ) ;
#25295=CARTESIAN_POINT ( 'NONE',  ( 23.41746824999999887, 0.6249999972688102812, 0.000000000000000000 ) ) ;
#25319=CARTESIAN_POINT ( 'NONE',  ( 24.50000000000000355, 3.849999994537637082, -7.960532557706203605 ) ) ;
#25331=CARTESIAN_POINT ( 'NONE',  ( 14.47279130897151767, 1.424999997268804997, -19.92008829642072598 ) ) ;
#25348=VECTOR ( 'NONE', #4518, 1000.000000000000000 ) ;
#25360=CARTESIAN_POINT ( 'NONE',  ( 24.50000000000000000, 17.99999999999998934, 0.000000000000000000 ) ) ;
#25365=LINE ( 'NONE', #30498, #27694 ) ;
#25369=CARTESIAN_POINT ( 'NONE',  ( -24.32582046900600758, 17.00000000000000000, -2.464910051867566843 ) ) ;
#25402=CARTESIAN_POINT ( 'NONE',  ( -4.523095164977116484E-15, 18.12499999726882649, 24.62258325217400312 ) ) ;
#25404=CARTESIAN_POINT ( 'NONE',  ( 0.000000000000000000, -20.99999999999998934, 0.000000000000000000 ) ) ;
#25429=CARTESIAN_POINT ( 'NONE',  ( 7.236395654485760609, 7.524999997268827734, -22.27133577429736633 ) ) ;
#25432=AXIS2_PLACEMENT_3D ( 'NONE', #23355, #2586, #23522 ) ;
#25446=CARTESIAN_POINT ( 'NONE',  ( 7.236395654485760609, 1.024999997268821739, -22.27133577429736633 ) ) ;
#25451=CARTESIAN_POINT ( 'NONE',  ( 19.82091636218621034, 7.800000000000001599, 14.40073868116559730 ) ) ;
#25455=CARTESIAN_POINT ( 'NONE',  ( -23.41746825000000243, 12.02499999726881974, -7.608796670333730638 ) ) ;
#25456=CARTESIAN_POINT ( 'NONE',  ( 18.94512977948576093, 0.8249999972688160099, -13.76444248337722875 ) ) ;
#25470=CARTESIAN_POINT ( 'NONE',  ( 14.47279130897151767, 2.924999997268815655, -19.92008829642072598 ) ) ;
#25472=ORIENTED_EDGE ( 'NONE', *, *, #29829, .T. ) ;
#25494=CARTESIAN_POINT ( 'NONE',  ( 7.570916362186207671, 13.34999999453762065, 23.30088464923126779 ) ) ;
#25514=ORIENTED_EDGE ( 'NONE', *, *, #2396, .F. ) ;
#25520=CARTESIAN_POINT ( 'NONE',  ( 7.570916362186207671, 9.599999999999997868, 23.30088464923126779 ) ) ;
#25540=CIRCLE ( 'NONE', #23342, 26.50000000000000355 ) ;
#25543=CARTESIAN_POINT ( 'NONE',  ( 7.236395654485760609, 15.02499999726880731, -22.27133577429736633 ) ) ;
#25546=CARTESIAN_POINT ( 'NONE',  ( 22.82331083168796582, 16.99999999999998934, 5.297087881879605220 ) ) ;
#25572=CARTESIAN_POINT ( 'NONE',  ( 7.570916362186207671, 13.34999999453762065, 23.30088464923126779 ) ) ;
#25576=CARTESIAN_POINT ( 'NONE',  ( -24.50000000000000000, 1.000000000000000888, -3.000384657911015469E-15 ) ) ;
#25591=CARTESIAN_POINT ( 'NONE',  ( 19.82091636218621389, 16.19999999999999218, -14.40073868116559197 ) ) ;
#25592=AXIS2_PLACEMENT_3D ( 'NONE', #33782, #13179, #5116 ) ;
#25599=AXIS2_PLACEMENT_3D ( 'NONE', #22410, #32858, #6958 ) ;
#25603=CARTESIAN_POINT ( 'NONE',  ( 23.41746824999999887, 5.224999997268801266, -7.608796670333727974 ) ) ;
#25610=DIRECTION ( 'NONE',  ( 0.000000000000000000, 0.000000000000000000, -1.000000000000000000 ) ) ;
#25618=CARTESIAN_POINT ( 'NONE',  ( -18.94512977948576093, 1.824999997268816898, 13.76444248337722698 ) ) ;
#25627=ORIENTED_EDGE ( 'NONE', *, *, #618, .F. ) ;
#25628=CARTESIAN_POINT ( 'NONE',  ( -18.94512977948576093, 10.32499999726882400, 13.76444248337722698 ) ) ;
#25629=CARTESIAN_POINT ( 'NONE',  ( -7.236395654485763274, 4.024999997268824181, 22.27133577429736633 ) ) ;
#25641=CARTESIAN_POINT ( 'NONE',  ( -23.41746825000000598, 7.724999997268809260, 7.608796670333726198 ) ) ;
#25662=CARTESIAN_POINT ( 'NONE',  ( -24.50000000000000000, 14.64999999453761603, -7.960532557706207157 ) ) ;
#25664=CARTESIAN_POINT ( 'NONE',  ( 7.570916362186207671, 15.34999999453762243, 23.30088464923126779 ) ) ;
#25676=CARTESIAN_POINT ( 'NONE',  ( -18.94512977948576093, 10.32499999726882400, 13.76444248337722698 ) ) ;
#25703=CARTESIAN_POINT ( 'NONE',  ( 7.570916362186213000, 16.39999999999999858, -23.30088464923126423 ) ) ;
#25715=DIRECTION ( 'NONE',  ( 0.000000000000000000, -1.000000000000000000, 0.000000000000000000 ) ) ;
#25742=CARTESIAN_POINT ( 'NONE',  ( 1.507698388325705758E-15, 15.12499999726880873, -24.62258325217400312 ) ) ;
#25767=CARTESIAN_POINT ( 'NONE',  ( -7.236395654485763274, 6.524999997268826846, 22.27133577429736633 ) ) ;
#25791=CARTESIAN_POINT ( 'NONE',  ( 14.47279130897151589, 10.82499999726882756, 19.92008829642072953 ) ) ;
#25792=CARTESIAN_POINT ( 'NONE',  ( -18.94512977948575738, 3.424999997268807217, -13.76444248337723231 ) ) ;
#25804=CARTESIAN_POINT ( 'NONE',  ( 14.47279130897151589, 10.32499999726881335, 19.92008829642072953 ) ) ;
#25827=CARTESIAN_POINT ( 'NONE',  ( -4.223320258572819786E-15, 15.24999999453762278, 24.50000000000000000 ) ) ;
#25829=CARTESIAN_POINT ( 'NONE',  ( -24.50000000000001066, 12.84999999453761532, 7.960532557706201828 ) ) ;
#25844=CARTESIAN_POINT ( 'NONE',  ( -7.236395654485763274, 10.52499999726880198, 22.27133577429736633 ) ) ;
#25849=ORIENTED_EDGE ( 'NONE', *, *, #609, .T. ) ;
#25851=ORIENTED_EDGE ( 'NONE', *, *, #31876, .T. ) ;
#25862=CARTESIAN_POINT ( 'NONE',  ( -15.14183272437242067, 4.699999999999996625, -20.84094480462497856 ) ) ;
#25911=CARTESIAN_POINT ( 'NONE',  ( -7.570916362186210335, 4.599999999999992539, -23.30088464923126779 ) ) ;
#25917=CYLINDRICAL_SURFACE ( 'NONE', #25432, 24.50000000000000000 ) ;
#25936=CARTESIAN_POINT ( 'NONE',  ( 7.236395654485755280, 6.724999997268804819, 22.27133577429736988 ) ) ;
#25962=CARTESIAN_POINT ( 'NONE',  ( 7.236395654485760609, 15.52499999726880731, -22.27133577429736633 ) ) ;
#25963=CARTESIAN_POINT ( 'NONE',  ( 14.47279130897151944, 4.924999997268811214, -19.92008829642072598 ) ) ;
#25977=CARTESIAN_POINT ( 'NONE',  ( 18.94512977948575738, 6.424999997268809437, 13.76444248337723408 ) ) ;
#25981=CARTESIAN_POINT ( 'NONE',  ( -3.712076227271900841E-14, 10.24999999453763344, -24.50000000000000000 ) ) ;
#25991=CARTESIAN_POINT ( 'NONE',  ( -15.14183272437242067, 6.449999994537612302, -20.84094480462497856 ) ) ;
#25996=CARTESIAN_POINT ( 'NONE',  ( -7.570916362186210335, 14.60000000000000142, -23.30088464923126779 ) ) ;
#26001=CARTESIAN_POINT ( 'NONE',  ( -19.82091636218621034, 10.54999999453762349, -14.40073868116559552 ) ) ;
#26009=CARTESIAN_POINT ( 'NONE',  ( 3.445340210940985210E-14, 7.249999994537622783, 24.50000000000000000 ) ) ;
#26018=CARTESIAN_POINT ( 'NONE',  ( 18.94512977948575738, 10.92499999726881299, 13.76444248337723408 ) ) ;
#26035=CARTESIAN_POINT ( 'NONE',  ( -24.50000000000000711, 5.100000000000012967, 7.960532557706201828 ) ) ;
#26055=FACE_OUTER_BOUND ( 'NONE', #16862, .T. ) ;
#26082=SHAPE_REPRESENTATION_RELATIONSHIP ( 'NONE' , 'NONE' ,  #33740, #13626 ) ;
#26085=CARTESIAN_POINT ( 'NONE',  ( -19.82091636218621034, 2.799999999999997158, -14.40073868116559552 ) ) ;
#26107=CARTESIAN_POINT ( 'NONE',  ( 18.94512977948576093, 11.32499999726882578, -13.76444248337722875 ) ) ;
#26118=FACE_OUTER_BOUND ( 'NONE', #6597, .T. ) ;
#26124=CARTESIAN_POINT ( 'NONE',  ( -7.236395654485763274, 4.024999997268824181, 22.27133577429736633 ) ) ;
#26134=CARTESIAN_POINT ( 'NONE',  ( 18.94512977948575738, 18.92499999726882010, 13.76444248337723408 ) ) ;
#26147=CARTESIAN_POINT ( 'NONE',  ( 7.236395654485760609, 11.02499999726880375, -22.27133577429736633 ) ) ;
#26176=CARTESIAN_POINT ( 'NONE',  ( 15.14183272437242245, 12.04999999453761106, -20.84094480462497856 ) ) ;
#26190=CARTESIAN_POINT ( 'NONE',  ( -7.236395654485757944, 7.724999997268805707, -22.27133577429736988 ) ) ;
#26226=CARTESIAN_POINT ( 'NONE',  ( 4.310114166470925490, 16.99999999999999289, -23.13846340751065611 ) ) ;
#26231=CARTESIAN_POINT ( 'NONE',  ( -15.14183272437242067, 12.44999999453762918, -20.84094480462497856 ) ) ;
#26238=ORIENTED_EDGE ( 'NONE', *, *, #29977, .T. ) ;
#26255=CARTESIAN_POINT ( 'NONE',  ( -24.50000000000000000, 3.000000000000002665, -3.000384657911015469E-15 ) ) ;
#26257=CARTESIAN_POINT ( 'NONE',  ( -19.82091636218621389, 2.949999994537627401, 14.40073868116558842 ) ) ;
#26272=CYLINDRICAL_SURFACE ( 'NONE', #33714, 15.00000000000000000 ) ;
#26278=CARTESIAN_POINT ( 'NONE',  ( 14.47279130897151944, 15.42499999726879878, -19.92008829642072598 ) ) ;
#26296=CARTESIAN_POINT ( 'NONE',  ( -23.41746825000000598, 5.724999997268815477, 7.608796670333726198 ) ) ;
#26305=CARTESIAN_POINT ( 'NONE',  ( 7.236395654485760609, 17.52499999726880731, -22.27133577429736633 ) ) ;
#26317=CARTESIAN_POINT ( 'NONE',  ( -23.41746825000000243, 11.52499999726880553, -7.608796670333730638 ) ) ;
#26338=CARTESIAN_POINT ( 'NONE',  ( -7.570916362186215665, 15.39999999999999680, 23.30088464923126423 ) ) ;
#26343=CARTESIAN_POINT ( 'NONE',  ( 1.507698388325705758E-15, 1.624999997268827823, -24.62258325217400312 ) ) ;
#26350=CARTESIAN_POINT ( 'NONE',  ( -7.570916362186210335, 6.599999999999994316, -23.30088464923126779 ) ) ;
#26357=CARTESIAN_POINT ( 'NONE',  ( -23.41746825000000243, 10.02499999726882507, -7.608796670333730638 ) ) ;
#26358=( BOUNDED_CURVE ( )  B_SPLINE_CURVE ( 2, ( #15881, #28736, #25996, #15716, #10894, #2827, #23432, #10384, #26508, #21367, #26338, #23769, #18116 ),
 .UNSPECIFIED., .F., .T. ) 
 B_SPLINE_CURVE_WITH_KNOTS ( ( 3, 2, 2, 2, 2, 2, 3 ),
 ( 0.8055555555555555802, 0.8111111111111111160, 0.8222222222222221877, 0.8333333333333333703, 0.8444444444444444420, 0.8555555555555555136, 0.8611111111111111605 ),
 .UNSPECIFIED. ) 
 CURVE ( )  GEOMETRIC_REPRESENTATION_ITEM ( )  RATIONAL_B_SPLINE_CURVE ( ( 0.9755282581475768211, 0.9755282581475768211, 1.000000000000000000, 0.9510565162951535312, 1.000000000000000000, 0.9510565162951535312, 1.000000000000000000, 0.9510565162951535312, 1.000000000000000000, 0.9510565162951535312, 1.000000000000000000, 0.9755282581475765991, 0.9755282581475768211 ) ) 
 REPRESENTATION_ITEM ( '' )  );
#26364=ORIENTED_EDGE ( 'NONE', *, *, #2863, .T. ) ;
#26423=CARTESIAN_POINT ( 'NONE',  ( -7.570916362186210335, 8.599999999999996092, -23.30088464923126779 ) ) ;
#26425=FACE_OUTER_BOUND ( 'NONE', #27241, .T. ) ;
#26432=CARTESIAN_POINT ( 'NONE',  ( 3.880418787951153803, 9.301254276084472750, 24.49999999999999645 ) ) ;
#26464=CARTESIAN_POINT ( 'NONE',  ( 7.236395654485760609, 5.024999997268825069, -22.27133577429736633 ) ) ;
#26473=CARTESIAN_POINT ( 'NONE',  ( -18.94512977948575738, 17.92499999726882010, -13.76444248337723231 ) ) ;
#26486=CARTESIAN_POINT ( 'NONE',  ( 23.41746825000000243, 18.52499999726881441, 7.608796670333735079 ) ) ;
#26488=EDGE_LOOP ( 'NONE', ( #14796, #25236, #31920, #14627 ) ) ;
#26508=CARTESIAN_POINT ( 'NONE',  ( -19.82091636218621389, 15.19999999999999218, 14.40073868116558842 ) ) ;
#26513=CARTESIAN_POINT ( 'NONE',  ( -23.41746824999999887, 2.124999997268811391, -2.867812753649727150E-15 ) ) ;
#26528=CARTESIAN_POINT ( 'NONE',  ( 14.47279130897151767, 13.42499999726880411, -19.92008829642072598 ) ) ;
#26529=ORIENTED_EDGE ( 'NONE', *, *, #9209, .F. ) ;
#26563=MECHANICAL_DESIGN_GEOMETRIC_PRESENTATION_REPRESENTATION('',(#1949),#30379);
#26574=VERTEX_POINT ( 'NONE', #28067 ) ;
#26592=CARTESIAN_POINT ( 'NONE',  ( -24.50000000000000355, 4.899999999999989697, -7.960532557706207157 ) ) ;
#26597=CARTESIAN_POINT ( 'NONE',  ( -14.47279130897151767, 5.324999997268826668, -19.92008829642072598 ) ) ;
#26615=CARTESIAN_POINT ( 'NONE',  ( 7.236395654485755280, 14.72499999726881192, 22.27133577429736988 ) ) ;
#26633=CARTESIAN_POINT ( 'NONE',  ( 1.507698388325705758E-15, 5.124999997268805174, -24.62258325217400312 ) ) ;
#26641=FACE_OUTER_BOUND ( 'NONE', #6343, .T. ) ;
#26654=CARTESIAN_POINT ( 'NONE',  ( -23.41746824999999887, 13.62499999726882116, -2.867812753649727150E-15 ) ) ;
#26655=CARTESIAN_POINT ( 'NONE',  ( 24.50000000000000000, 14.00000000000001243, 0.000000000000000000 ) ) ;
#26666=CARTESIAN_POINT ( 'NONE',  ( -7.570916362186215665, 3.149999994537633352, 23.30088464923126423 ) ) ;
#26681=CARTESIAN_POINT ( 'NONE',  ( -18.94512977948575738, 1.924999997268805885, -13.76444248337723231 ) ) ;
#26694=CARTESIAN_POINT ( 'NONE',  ( -23.41746824999999887, 16.12499999726882294, -2.867812753649727150E-15 ) ) ;
#26720=CARTESIAN_POINT ( 'NONE',  ( -24.50000000000000000, 10.90000000000000568, -7.960532557706207157 ) ) ;
#26739=CARTESIAN_POINT ( 'NONE',  ( -19.82091636218621389, 13.19999999999998863, 14.40073868116558842 ) ) ;
#26759=CARTESIAN_POINT ( 'NONE',  ( 15.14183272437241889, 9.699999999999985079, 20.84094480462498211 ) ) ;
#26761=CARTESIAN_POINT ( 'NONE',  ( -24.50000000000000355, 8.649999994537630243, -7.960532557706207157 ) ) ;
#26763=CARTESIAN_POINT ( 'NONE',  ( 7.236395654485760609, 7.024999997268826846, -22.27133577429736633 ) ) ;
#26764=EDGE_CURVE ( 'NONE', #29527, #24126, #10011, .T. ) ;
#26782=CARTESIAN_POINT ( 'NONE',  ( -23.41746825000000243, 16.22499999726880304, 7.608796670333725309 ) ) ;
#26797=CARTESIAN_POINT ( 'NONE',  ( -7.236395654485763274, 2.024999997268822405, 22.27133577429736633 ) ) ;
#26805=CARTESIAN_POINT ( 'NONE',  ( -4.223320258572819786E-15, 13.50000000000000355, 24.50000000000000000 ) ) ;
#26818=CARTESIAN_POINT ( 'NONE',  ( 23.41746825000000243, 16.52499999726882152, 7.608796670333735079 ) ) ;
#26842=CARTESIAN_POINT ( 'NONE',  ( -4.523095164977116484E-15, 2.624999997268825158, 24.62258325217400312 ) ) ;
#26856=DIRECTION ( 'NONE',  ( 0.000000000000000000, -1.000000000000000000, 0.000000000000000000 ) ) ;
#26859=CARTESIAN_POINT ( 'NONE',  ( 1.507698388325705758E-15, 15.62499999726882116, -24.62258325217400312 ) ) ;
#26882=CARTESIAN_POINT ( 'NONE',  ( 7.313012447739250820E-14, 11.49999999999999112, 24.50000000000000000 ) ) ;
#26889=CARTESIAN_POINT ( 'NONE',  ( 9.103978835402296355, 16.99999999999999645, 22.05180196682243832 ) ) ;
#26919=CARTESIAN_POINT ( 'NONE',  ( -19.82091636218621034, 14.80000000000000782, -14.40073868116559552 ) ) ;
#26922=CARTESIAN_POINT ( 'NONE',  ( 14.47279130897151767, 10.32499999726881335, 19.92008829642072953 ) ) ;
#26923=CARTESIAN_POINT ( 'NONE',  ( 19.82091636218621389, 4.200000000000009059, -14.40073868116559197 ) ) ;
#26935=CARTESIAN_POINT ( 'NONE',  ( -7.579748464070165821E-14, 16.50000000000000355, -24.50000000000000000 ) ) ;
#26954=CARTESIAN_POINT ( 'NONE',  ( -23.41746825000000598, 13.72499999726882258, 7.608796670333726198 ) ) ;
#26975=CARTESIAN_POINT ( 'NONE',  ( -14.47279130897152122, 15.92499999726881121, 19.92008829642072243 ) ) ;
#26980=CARTESIAN_POINT ( 'NONE',  ( 3.000384657911015469E-15, 16.99999999999998579, 24.50000000000000000 ) ) ;
#26989=CARTESIAN_POINT ( 'NONE',  ( -7.570916362186210335, 2.349999994537638415, -23.30088464923126779 ) ) ;
#26994=FACE_OUTER_BOUND ( 'NONE', #31134, .T. ) ;
#26997=PRESENTATION_STYLE_ASSIGNMENT (( #29727 ) ) ;
#27003=CARTESIAN_POINT ( 'NONE',  ( 7.236395654485760609, 3.524999997268824181, -22.27133577429736633 ) ) ;
#27022=CARTESIAN_POINT ( 'NONE',  ( 14.47279130897151589, 16.82499999726881512, 19.92008829642072953 ) ) ;
#27046=AXIS2_PLACEMENT_3D ( 'NONE', #33786, #10784, #30855 ) ;
#27063=CARTESIAN_POINT ( 'NONE',  ( -3.880418787951142701, 13.44874571845315536, 24.49999999999999645 ) ) ;
#27069=EDGE_LOOP ( 'NONE', ( #516, #12939, #32872, #13113 ) ) ;
#27088=CARTESIAN_POINT ( 'NONE',  ( 7.570916362186207671, 13.60000000000000142, 23.30088464923126779 ) ) ;
#27092=CARTESIAN_POINT ( 'NONE',  ( -7.236395654485763274, 8.024999997268828622, 22.27133577429736633 ) ) ;
#27127=CARTESIAN_POINT ( 'NONE',  ( -23.41746825000000598, 11.72499999726880127, 7.608796670333726198 ) ) ;
#27148=CARTESIAN_POINT ( 'NONE',  ( -14.47279130897151589, 17.32499999726879381, -19.92008829642072598 ) ) ;
#27152=CARTESIAN_POINT ( 'NONE',  ( -14.47279130897151767, 3.824999997268816454, -19.92008829642072598 ) ) ;
#27175=CARTESIAN_POINT ( 'NONE',  ( -23.41746825000000243, 4.024999997268810858, -7.608796670333730638 ) ) ;
#27192=CARTESIAN_POINT ( 'NONE',  ( 1.507698388325705758E-15, 13.62499999726882827, -24.62258325217400312 ) ) ;
#27216=CARTESIAN_POINT ( 'NONE',  ( -24.50000000000000000, 16.74999999453763522, -3.000384657911015469E-15 ) ) ;
#27232=CARTESIAN_POINT ( 'NONE',  ( 0.000000000000000000, -20.99999999999998934, 0.000000000000000000 ) ) ;
#27241=EDGE_LOOP ( 'NONE', ( #27533, #14366, #8941, #27537, #10029, #28131, #15952, #14127, #17891, #11351, #3858, #30911, #4362, #2062, #25627, #12857, #12215, #16327, #18147 ) ) ;
#27258=CARTESIAN_POINT ( 'NONE',  ( -24.50000000000001066, 15.09999999999998899, 7.960532557706201828 ) ) ;
#27262=CARTESIAN_POINT ( 'NONE',  ( 23.41746824999999887, 10.52499999726880731, 7.608796670333735079 ) ) ;
#27263=CARTESIAN_POINT ( 'NONE',  ( -24.50000000000000711, 9.100000000000003197, 7.960532557706201828 ) ) ;
#27296=CARTESIAN_POINT ( 'NONE',  ( 7.236395654485755280, 10.22499999726880837, 22.27133577429736988 ) ) ;
#27312=( BOUNDED_CURVE ( )  B_SPLINE_CURVE ( 2, ( #24133, #935, #21561, #21393, #11414, #1095, #21890, #13502, #11091, #32340, #18821, #19317, #6265 ),
 .UNSPECIFIED., .F., .F. ) 
 B_SPLINE_CURVE_WITH_KNOTS ( ( 3, 2, 2, 2, 2, 2, 3 ),
 ( 0.02777777777777777971, 0.03333333333333333287, 0.04444444444444444614, 0.05555555555555555247, 0.06666666666666667962, 0.07777777777777777901, 0.08333333333333334259 ),
 .UNSPECIFIED. ) 
 CURVE ( )  GEOMETRIC_REPRESENTATION_ITEM ( )  RATIONAL_B_SPLINE_CURVE ( ( 0.9755282581475768211, 0.9755282581475768211, 1.000000000000000000, 0.9510565162951535312, 1.000000000000000000, 0.9510565162951535312, 1.000000000000000000, 0.9510565162951535312, 1.000000000000000000, 0.9510565162951535312, 1.000000000000000000, 0.9755282581475767101, 0.9755282581475768211 ) ) 
 REPRESENTATION_ITEM ( '' )  );
#27325=CARTESIAN_POINT ( 'NONE',  ( -7.236395654485763274, 4.524999997268825069, 22.27133577429736633 ) ) ;
#27329=ORIENTED_EDGE ( 'NONE', *, *, #32821, .T. ) ;
#27330=EDGE_LOOP ( 'NONE', ( #8107, #20684, #15353, #910 ) ) ;
#27347=CARTESIAN_POINT ( 'NONE',  ( 14.47279130897151589, 6.824999997268808904, 19.92008829642072953 ) ) ;
#27362=CARTESIAN_POINT ( 'NONE',  ( 1.507698388325705758E-15, 5.124999997268805174, -24.62258325217400312 ) ) ;
#27384=CARTESIAN_POINT ( 'NONE',  ( 24.50000000000000355, 7.649999994537632908, 7.960532557706212486 ) ) ;
#27391=CARTESIAN_POINT ( 'NONE',  ( -2.361898896031838557, 16.99999999999998579, 24.02576800177196503 ) ) ;
#27393=CARTESIAN_POINT ( 'NONE',  ( 3.880418787951132042, 2.448745718453165576, -24.50000000000000355 ) ) ;
#27412=CARTESIAN_POINT ( 'NONE',  ( 3.880418787951140036, 16.19874571299077459, -24.49999999999999645 ) ) ;
#27425=CARTESIAN_POINT ( 'NONE',  ( 24.50000000000000000, 10.00000000000000888, 0.000000000000000000 ) ) ;
#27429=CARTESIAN_POINT ( 'NONE',  ( 14.47279130897151944, 12.92499999726881832, -19.92008829642072598 ) ) ;
#27447=( BOUNDED_CURVE ( )  B_SPLINE_CURVE ( 2, ( #11476, #24521, #21789, #16145, #19049, #21622, #29488, #3419, #26923, #8730, #29650, #5662, #991 ),
 .UNSPECIFIED., .F., .F. ) 
 B_SPLINE_CURVE_WITH_KNOTS ( ( 3, 2, 2, 2, 2, 2, 3 ),
 ( 0.1944444444444444475, 0.2000000000000000111, 0.2111111111111111105, 0.2222222222222222099, 0.2333333333333333370, 0.2444444444444444364, 0.2500000000000000000 ),
 .UNSPECIFIED. ) 
 CURVE ( )  GEOMETRIC_REPRESENTATION_ITEM ( )  RATIONAL_B_SPLINE_CURVE ( ( 0.9755282581475768211, 0.9755282581475768211, 1.000000000000000000, 0.9510565162951535312, 1.000000000000000000, 0.9510565162951535312, 1.000000000000000000, 0.9510565162951535312, 1.000000000000000000, 0.9510565162951535312, 1.000000000000000000, 0.9755282581475767101, 0.9755282581475768211 ) ) 
 REPRESENTATION_ITEM ( '' )  );
#27460=DIRECTION ( 'NONE',  ( 0.000000000000000000, 0.000000000000000000, 1.000000000000000000 ) ) ;
#27463=CARTESIAN_POINT ( 'NONE',  ( 18.94512977948575738, 10.42499999726881299, 13.76444248337723408 ) ) ;
#27489=CARTESIAN_POINT ( 'NONE',  ( 14.47279130897151767, 2.824999997268819119, 19.92008829642072953 ) ) ;
#27492=ORIENTED_EDGE ( 'NONE', *, *, #16924, .T. ) ;
#27505=CARTESIAN_POINT ( 'NONE',  ( 3.000384657911015469E-15, 16.99999999999998579, 24.50000000000000000 ) ) ;
#27508=CARTESIAN_POINT ( 'NONE',  ( 0.000000000000000000, -22.99999999999999289, -15.00000000000000000 ) ) ;
#27513=CARTESIAN_POINT ( 'NONE',  ( 23.41746825000000243, 5.024999997268808194, 7.608796670333735079 ) ) ;
#27526=CARTESIAN_POINT ( 'NONE',  ( -7.236395654485763274, 18.52499999726881086, 22.27133577429736633 ) ) ;
#27533=ORIENTED_EDGE ( 'NONE', *, *, #24344, .T. ) ;
#27537=ORIENTED_EDGE ( 'NONE', *, *, #24981, .F. ) ;
#27551=CARTESIAN_POINT ( 'NONE',  ( -24.50000000000000355, 4.649999994537640902, -7.960532557706207157 ) ) ;
#27566=CARTESIAN_POINT ( 'NONE',  ( -23.41746825000000598, 2.224999997268808816, 7.608796670333726198 ) ) ;
#27592=CARTESIAN_POINT ( 'NONE',  ( -15.14183272437242600, 17.30000000000000782, 20.84094480462497856 ) ) ;
#27596=CARTESIAN_POINT ( 'NONE',  ( -18.94512977948575738, 11.42499999726881477, -13.76444248337723231 ) ) ;
#27597=EDGE_CURVE ( 'NONE', #5367, #4913, #32122, .T. ) ;
#27600=CARTESIAN_POINT ( 'NONE',  ( -21.69117583031640351, 16.99999999999999289, -10.83878137934375374 ) ) ;
#27625=LINE ( 'NONE', #32920, #5901 ) ;
#27635=CARTESIAN_POINT ( 'NONE',  ( -18.94512977948576093, 9.824999997268824004, 13.76444248337722698 ) ) ;
#27659=CARTESIAN_POINT ( 'NONE',  ( 18.94512977948576093, 1.324999997268816454, -13.76444248337722875 ) ) ;
#27676=( NAMED_UNIT ( * ) SI_UNIT ( $, .STERADIAN. ) SOLID_ANGLE_UNIT ( ) );
#27683=CARTESIAN_POINT ( 'NONE',  ( 23.41746824999999887, 5.124999997268814056, 0.000000000000000000 ) ) ;
#27694=VECTOR ( 'NONE', #8355, 1000.000000000000000 ) ;
#27696=CARTESIAN_POINT ( 'NONE',  ( -23.41746825000000598, 5.724999997268815477, 7.608796670333726198 ) ) ;
#27723=CARTESIAN_POINT ( 'NONE',  ( -15.14183272437242600, 7.049999994537622605, 20.84094480462497856 ) ) ;
#27731=CARTESIAN_POINT ( 'NONE',  ( 7.570916362186213000, 2.400000000000013234, -23.30088464923126423 ) ) ;
#27749=CARTESIAN_POINT ( 'NONE',  ( -7.570916362186215665, 3.399999999999986144, 23.30088464923126423 ) ) ;
#27765=CARTESIAN_POINT ( 'NONE',  ( 19.82091636218621389, 16.19999999999999218, -14.40073868116559197 ) ) ;
#27806=CARTESIAN_POINT ( 'NONE',  ( 7.570916362186213000, 0.4000000000000114575, -23.30088464923126423 ) ) ;
#27858=CARTESIAN_POINT ( 'NONE',  ( 14.47279130897151589, 4.824999997268814234, 19.92008829642072953 ) ) ;
#27871=CARTESIAN_POINT ( 'NONE',  ( 23.41746825000000243, 19.02499999726880375, 7.608796670333735079 ) ) ;
#27895=CARTESIAN_POINT ( 'NONE',  ( -19.82091636218621389, 6.949999994537630954, 14.40073868116558842 ) ) ;
#27937=CARTESIAN_POINT ( 'NONE',  ( 19.82091636218621034, 15.80000000000000782, 14.40073868116559730 ) ) ;
#27938=ADVANCED_FACE ( 'NONE', ( #2438 ), #15832, .T. ) ;
#27943=CARTESIAN_POINT ( 'NONE',  ( 23.41746824999999887, 14.52499999726882685, 7.608796670333735079 ) ) ;
#27947=CARTESIAN_POINT ( 'NONE',  ( 21.93819159779297223, 16.99999999999998934, 8.226848600189008209 ) ) ;
#27958=VERTEX_POINT ( 'NONE', #15318 ) ;
#27976=CARTESIAN_POINT ( 'NONE',  ( 7.236395654485755280, 18.22499999726881370, 22.27133577429736988 ) ) ;
#27991=CARTESIAN_POINT ( 'NONE',  ( 15.14183272437242422, 6.300000000000004263, -20.84094480462497856 ) ) ;
#28000=CARTESIAN_POINT ( 'NONE',  ( 23.41746824999999887, 7.124999997268815832, 0.000000000000000000 ) ) ;
#28001=VERTEX_POINT ( 'NONE', #15666 ) ;
#28007=ORIENTED_EDGE ( 'NONE', *, *, #11255, .F. ) ;
#28019=CARTESIAN_POINT ( 'NONE',  ( 15.14183272437242067, 7.699999999999988631, 20.84094480462498211 ) ) ;
#28023=CARTESIAN_POINT ( 'NONE',  ( -14.47279130897152122, 16.42499999726882365, 19.92008829642072243 ) ) ;
#28030=CARTESIAN_POINT ( 'NONE',  ( 0.000000000000000000, 16.99999999999998579, -24.50000000000000000 ) ) ;
#28039=CARTESIAN_POINT ( 'NONE',  ( -18.94512977948575738, 3.424999997268807217, -13.76444248337723231 ) ) ;
#28063=CARTESIAN_POINT ( 'NONE',  ( -24.50000000000000000, 10.74999999453762811, -3.000384657911015469E-15 ) ) ;
#28067=CARTESIAN_POINT ( 'NONE',  ( 7.313012447739250820E-14, 11.49999999999999112, 24.50000000000000000 ) ) ;
#28071=CARTESIAN_POINT ( 'NONE',  ( 0.000000000000000000, -20.99999999999998934, 0.000000000000000000 ) ) ;
#28097=CARTESIAN_POINT ( 'NONE',  ( -19.82091636218621389, 5.200000000000009948, 14.40073868116558842 ) ) ;
#28111=CARTESIAN_POINT ( 'NONE',  ( -18.94512977948576093, 13.82499999726879913, 13.76444248337722698 ) ) ;
#28114=CARTESIAN_POINT ( 'NONE',  ( -24.50000000000000000, 4.749999994537623671, -3.000384657911015469E-15 ) ) ;
#28122=CARTESIAN_POINT ( 'NONE',  ( 24.50000000000000000, 0.8749999972688105032, 0.000000000000000000 ) ) ;
#28129=EDGE_CURVE ( 'NONE', #6559, #11786, #348, .T. ) ;
#28131=ORIENTED_EDGE ( 'NONE', *, *, #31174, .F. ) ;
#28144=FILL_AREA_STYLE_COLOUR ( '', #21157 ) ;
#28147=CARTESIAN_POINT ( 'NONE',  ( -14.47279130897152122, 17.92499999726880588, 19.92008829642072243 ) ) ;
#28149=DIRECTION ( 'NONE',  ( 0.000000000000000000, -1.000000000000000000, 0.000000000000000000 ) ) ;
#28162=CARTESIAN_POINT ( 'NONE',  ( 1.555960095263670572E-15, 6.499999999999994671, -24.50000000000000000 ) ) ;
#28171=CARTESIAN_POINT ( 'NONE',  ( 23.41746824999999887, 11.02499999726882152, 7.608796670333735079 ) ) ;
#28172=ORIENTED_EDGE ( 'NONE', *, *, #24060, .F. ) ;
#28179=CARTESIAN_POINT ( 'NONE',  ( 19.82091636218621034, 5.549999994537619052, 14.40073868116559730 ) ) ;
#28186=CARTESIAN_POINT ( 'NONE',  ( -23.41746824999999887, 1.624999997268811169, -2.867812753649727150E-15 ) ) ;
#28195=CARTESIAN_POINT ( 'NONE',  ( 18.94512977948575738, 12.92499999726881654, 13.76444248337723408 ) ) ;
#28196=CARTESIAN_POINT ( 'NONE',  ( -14.47279130897152299, 5.924999997268808549, 19.92008829642072243 ) ) ;
#28210=CARTESIAN_POINT ( 'NONE',  ( 7.236395654485755280, 12.22499999726881015, 22.27133577429736988 ) ) ;
#28234=CARTESIAN_POINT ( 'NONE',  ( 19.82091636218621389, 15.94999999453763984, -14.40073868116559197 ) ) ;
#28249=CARTESIAN_POINT ( 'NONE',  ( -3.880418787951142701, 11.19874571299077637, 24.49999999999999645 ) ) ;
#28282=CYLINDRICAL_SURFACE ( 'NONE', #3039, 24.50000000000000000 ) ;
#28289=CARTESIAN_POINT ( 'NONE',  ( 7.313012447739250820E-14, 13.24999999453762456, 24.50000000000000000 ) ) ;
#28296=VERTEX_POINT ( 'NONE', #21648 ) ;
#28300=ORIENTED_EDGE ( 'NONE', *, *, #10286, .T. ) ;
#28310=CARTESIAN_POINT ( 'NONE',  ( 19.82091636218621034, 13.54999999453762527, 14.40073868116559730 ) ) ;
#28314=CARTESIAN_POINT ( 'NONE',  ( -23.41746825000000243, 17.52499999726881796, -7.608796670333730638 ) ) ;
#28331=CARTESIAN_POINT ( 'NONE',  ( 19.82091636218621389, 6.200000000000010836, -14.40073868116559197 ) ) ;
#28332=VECTOR ( 'NONE', #29872, 1000.000000000000000 ) ;
#28338=CARTESIAN_POINT ( 'NONE',  ( 3.880418787951139148, 0.4487457184531665200, -24.50000000000000000 ) ) ;
#28343=CARTESIAN_POINT ( 'NONE',  ( -14.47279130897151767, 9.824999997268800911, -19.92008829642072598 ) ) ;
#28367=ORIENTED_EDGE ( 'NONE', *, *, #7482, .T. ) ;
#28368=CARTESIAN_POINT ( 'NONE',  ( -14.47279130897152122, 10.42499999726881299, 19.92008829642072243 ) ) ;
#28369=CARTESIAN_POINT ( 'NONE',  ( -23.41746825000000243, 3.724999997268820362, 7.608796670333725309 ) ) ;
#28381=CARTESIAN_POINT ( 'NONE',  ( -23.41746825000000598, 9.724999997268804819, 7.608796670333726198 ) ) ;
#28404=CARTESIAN_POINT ( 'NONE',  ( -24.50000000000001066, 10.84999999453761887, 7.960532557706201828 ) ) ;
#28418=CARTESIAN_POINT ( 'NONE',  ( 18.94512977948576093, 9.324999997268824004, -13.76444248337722875 ) ) ;
#28430=CARTESIAN_POINT ( 'NONE',  ( -7.570916362186210335, 2.599999999999991207, -23.30088464923126779 ) ) ;
#28453=DIRECTION ( 'NONE',  ( 0.000000000000000000, 0.000000000000000000, -1.000000000000000000 ) ) ;
#28482=CARTESIAN_POINT ( 'NONE',  ( 7.570916362186207671, 7.599999999999996092, 23.30088464923126779 ) ) ;
#28484=CARTESIAN_POINT ( 'NONE',  ( 1.577395562988744260E-15, 2.249999994537629444, -25.76082449383753925 ) ) ;
#28493=CARTESIAN_POINT ( 'NONE',  ( 15.14183272437242422, 16.30000000000000782, -20.84094480462497856 ) ) ;
#28502=CARTESIAN_POINT ( 'NONE',  ( 14.47279130897151944, 5.424999997268823648, -19.92008829642072598 ) ) ;
#28510=ADVANCED_FACE ( 'NONE', ( #33011 ), #32349, .T. ) ;
#28512=CARTESIAN_POINT ( 'NONE',  ( 24.50000000000000000, 5.849999994537632197, -7.960532557706203605 ) ) ;
#28530=CARTESIAN_POINT ( 'NONE',  ( -7.236395654485763274, 14.52499999726880553, 22.27133577429736633 ) ) ;
#28531=CARTESIAN_POINT ( 'NONE',  ( -14.47279130897152299, 3.924999997268813878, 19.92008829642072243 ) ) ;
#28542=CARTESIAN_POINT ( 'NONE',  ( 18.94512977948575738, 10.42499999726881299, 13.76444248337723408 ) ) ;
#28544=ORIENTED_EDGE ( 'NONE', *, *, #20704, .T. ) ;
#28568=CARTESIAN_POINT ( 'NONE',  ( 24.50000000000000355, 13.64999999453761781, 7.960532557706212486 ) ) ;
#28583=CARTESIAN_POINT ( 'NONE',  ( 18.94512977948575738, 6.924999997268810326, 13.76444248337723408 ) ) ;
#28605=CARTESIAN_POINT ( 'NONE',  ( 0.000000000000000000, 16.99999999999998579, -24.50000000000000000 ) ) ;
#28619=CARTESIAN_POINT ( 'NONE',  ( 0.000000000000000000, -22.99999999999999289, 0.000000000000000000 ) ) ;
#28622=CARTESIAN_POINT ( 'NONE',  ( -24.50000000000000000, 12.64999999453762136, -7.960532557706207157 ) ) ;
#28623=DIRECTION ( 'NONE',  ( 0.000000000000000000, -1.000000000000000000, 0.000000000000000000 ) ) ;
#28629=ORIENTED_EDGE ( 'NONE', *, *, #19434, .T. ) ;
#28650=CARTESIAN_POINT ( 'NONE',  ( 15.14183272437242245, 8.300000000000000711, -20.84094480462497856 ) ) ;
#28665=DIRECTION ( 'NONE',  ( 0.000000000000000000, -1.000000000000000000, 0.000000000000000000 ) ) ;
#28677=CARTESIAN_POINT ( 'NONE',  ( 23.41746824999999887, 7.024999997268802865, 7.608796670333735079 ) ) ;
#28685=CARTESIAN_POINT ( 'NONE',  ( -4.223320258572819786E-15, 5.249999994537629888, 24.50000000000000000 ) ) ;
#28687=DIRECTION ( 'NONE',  ( -0.000000000000000000, -1.000000000000000000, -0.000000000000000000 ) ) ;
#28694=CARTESIAN_POINT ( 'NONE',  ( -23.41746825000000598, 3.724999997268819918, 7.608796670333726198 ) ) ;
#28703=CARTESIAN_POINT ( 'NONE',  ( -18.94512977948576093, 12.32499999726879913, 13.76444248337722698 ) ) ;
#28716=CARTESIAN_POINT ( 'NONE',  ( -4.523095164977116484E-15, 10.12499999726881938, 24.62258325217400312 ) ) ;
#28724=ORIENTED_EDGE ( 'NONE', *, *, #15463, .T. ) ;
#28727=ORIENTED_EDGE ( 'NONE', *, *, #2396, .T. ) ;
#28736=CARTESIAN_POINT ( 'NONE',  ( -3.880418787951136483, 14.55125428154684997, -24.50000000000000000 ) ) ;
#28741=CARTESIAN_POINT ( 'NONE',  ( 24.50000000000000355, 9.849999994537622428, -7.960532557706203605 ) ) ;
#28757=CARTESIAN_POINT ( 'NONE',  ( -23.41746825000000243, 8.024999997268801977, -7.608796670333730638 ) ) ;
#28795=LINE ( 'NONE', #33787, #21520 ) ;
#28821=CARTESIAN_POINT ( 'NONE',  ( 7.570916362186213000, 4.399999999999987033, -23.30088464923126423 ) ) ;
#28829=CARTESIAN_POINT ( 'NONE',  ( 7.570916362186213000, 10.14999999453763913, -23.30088464923126423 ) ) ;
#28832=CARTESIAN_POINT ( 'NONE',  ( 0.000000000000000000, -22.99999999999999289, -26.50000000000000355 ) ) ;
#28833=CARTESIAN_POINT ( 'NONE',  ( 3.000384657911015469E-15, 16.99999999999998579, 24.50000000000000000 ) ) ;
#28844=CARTESIAN_POINT ( 'NONE',  ( -18.94512977948575738, 11.92499999726881477, -13.76444248337723231 ) ) ;
#28862=CARTESIAN_POINT ( 'NONE',  ( -4.523095164977116484E-15, 2.124999997268812280, 24.62258325217400312 ) ) ;
#28872=CARTESIAN_POINT ( 'NONE',  ( -7.236395654485763274, 18.52499999726881086, 22.27133577429736633 ) ) ;
#28884=CARTESIAN_POINT ( 'NONE',  ( 23.41746824999999887, 6.624999997268815832, 0.000000000000000000 ) ) ;
#28896=VECTOR ( 'NONE', #21278, 1000.000000000000000 ) ;
#28897=CARTESIAN_POINT ( 'NONE',  ( -24.50000000000000000, 6.749999994537625447, -3.000384657911015469E-15 ) ) ;
#28907=CARTESIAN_POINT ( 'NONE',  ( -19.82091636218621389, 16.94999999453764161, 14.40073868116558842 ) ) ;
#28917=CARTESIAN_POINT ( 'NONE',  ( 1.836970198721029589E-15, -22.99999999999999289, 15.00000000000000000 ) ) ;
#28922=CARTESIAN_POINT ( 'NONE',  ( 14.47279130897151589, 6.824999997268808904, 19.92008829642072953 ) ) ;
#28952=CIRCLE ( 'NONE', #19616, 26.50000000000000355 ) ;
#28989=CARTESIAN_POINT ( 'NONE',  ( -15.14183272437242600, 5.300000000000006928, 20.84094480462497856 ) ) ;
#28997=CARTESIAN_POINT ( 'NONE',  ( 0.000000000000000000, -20.99999999999998934, -26.50000000000000355 ) ) ;
#29011=CARTESIAN_POINT ( 'NONE',  ( -23.41746824999999887, 16.12499999726882294, -2.867812753649727150E-15 ) ) ;
#29026=CARTESIAN_POINT ( 'NONE',  ( -4.523095164977116484E-15, 4.124999997268806951, 24.62258325217400312 ) ) ;
#29035=CARTESIAN_POINT ( 'NONE',  ( 18.94512977948576093, 17.32499999726880446, -13.76444248337722875 ) ) ;
#29047=CARTESIAN_POINT ( 'NONE',  ( 14.47279130897151767, 16.92499999726880944, -19.92008829642072598 ) ) ;
#29073=CARTESIAN_POINT ( 'NONE',  ( 23.41746824999999887, 1.124999997268810725, 0.000000000000000000 ) ) ;
#29085=CARTESIAN_POINT ( 'NONE',  ( 3.445340210940985210E-14, 7.499999999999994671, 24.50000000000000000 ) ) ;
#29087=CARTESIAN_POINT ( 'NONE',  ( -18.94512977948576093, 8.324999997268822227, 13.76444248337722698 ) ) ;
#29124=LINE ( 'NONE', #5959, #20189 ) ;
#29150=CARTESIAN_POINT ( 'NONE',  ( 1.577395562988744260E-15, 4.500000000000003553, -25.76082449383753925 ) ) ;
#29155=CARTESIAN_POINT ( 'NONE',  ( -14.47279130897152299, 1.924999997268818541, 19.92008829642072243 ) ) ;
#29156=CARTESIAN_POINT ( 'NONE',  ( -19.82091636218621389, 9.200000000000013500, 14.40073868116558842 ) ) ;
#29178=CARTESIAN_POINT ( 'NONE',  ( -18.94512977948576093, 14.32499999726880091, 13.76444248337722698 ) ) ;
#29194=CARTESIAN_POINT ( 'NONE',  ( -18.94512977948576093, 7.824999997268822227, 13.76444248337722698 ) ) ;
#29216=CARTESIAN_POINT ( 'NONE',  ( 7.236395654485760609, 15.02499999726880731, -22.27133577429736633 ) ) ;
#29223=ORIENTED_EDGE ( 'NONE', *, *, #19113, .F. ) ;
#29242=CARTESIAN_POINT ( 'NONE',  ( 14.47279130897151767, 3.424999997268800112, -19.92008829642072598 ) ) ;
#29256=CARTESIAN_POINT ( 'NONE',  ( -7.236395654485763274, 12.52499999726880375, 22.27133577429736633 ) ) ;
#29311=CARTESIAN_POINT ( 'NONE',  ( 3.245314017740486554E-15, -20.99999999999998934, 26.50000000000000355 ) ) ;
#29322=CARTESIAN_POINT ( 'NONE',  ( 19.82091636218621389, 14.19999999999999041, -14.40073868116559197 ) ) ;
#29324=CARTESIAN_POINT ( 'NONE',  ( -15.14183272437241889, 4.449999994537617631, -20.84094480462497856 ) ) ;
#29327=CARTESIAN_POINT ( 'NONE',  ( 23.41746824999999887, 6.724999997268811924, -7.608796670333727974 ) ) ;
#29328=CARTESIAN_POINT ( 'NONE',  ( -3.880418787951142701, 9.448745718453144704, 24.49999999999999645 ) ) ;
#29346=CARTESIAN_POINT ( 'NONE',  ( -23.41746825000000243, 14.22499999726880837, 7.608796670333725309 ) ) ;
#29362=CARTESIAN_POINT ( 'NONE',  ( 23.41746825000000243, 2.524999997268798868, 7.608796670333735079 ) ) ;
#29372=CARTESIAN_POINT ( 'NONE',  ( 18.94512977948575738, 16.92499999726882010, 13.76444248337723408 ) ) ;
#29386=CARTESIAN_POINT ( 'NONE',  ( -18.94512977948575738, 15.42499999726881832, -13.76444248337723231 ) ) ;
#29387=CARTESIAN_POINT ( 'NONE',  ( 3.880418787951140036, 14.44874571845315536, -24.49999999999999645 ) ) ;
#29401=CARTESIAN_POINT ( 'NONE',  ( 0.000000000000000000, 16.99999999999998579, 0.000000000000000000 ) ) ;
#29410=CARTESIAN_POINT ( 'NONE',  ( -19.82091636218621034, 16.54999999453762882, -14.40073868116559552 ) ) ;
#29425=CARTESIAN_POINT ( 'NONE',  ( -23.41746825000000243, 12.02499999726881974, -7.608796670333730638 ) ) ;
#29426=EDGE_LOOP ( 'NONE', ( #14267, #20599, #32962, #1199 ) ) ;
#29457=CARTESIAN_POINT ( 'NONE',  ( 3.880418787951134707, 11.30125427608447097, 24.50000000000000000 ) ) ;
#29483=CARTESIAN_POINT ( 'NONE',  ( 15.14183272437241889, 13.70000000000000462, 20.84094480462498211 ) ) ;
#29487=CARTESIAN_POINT ( 'NONE',  ( 18.94512977948576093, 10.82499999726882578, -13.76444248337722875 ) ) ;
#29488=CARTESIAN_POINT ( 'NONE',  ( 24.50000000000000000, 4.000000000000003553, 0.000000000000000000 ) ) ;
#29491=CARTESIAN_POINT ( 'NONE',  ( 23.37900124392997014, 16.99999999999998934, -1.544069416992833066 ) ) ;
#29493=PRODUCT_DEFINITION_CONTEXT ( 'detailed design', #7454, 'design' ) ;
#29506=CARTESIAN_POINT ( 'NONE',  ( -7.236395654485763274, 16.52499999726880731, 22.27133577429736633 ) ) ;
#29520=CARTESIAN_POINT ( 'NONE',  ( 23.41746825000000243, 12.72499999726882436, -7.608796670333727974 ) ) ;
#29527=VERTEX_POINT ( 'NONE', #31061 ) ;
#29540=CARTESIAN_POINT ( 'NONE',  ( 14.47279130897151589, 16.32499999726882933, 19.92008829642072953 ) ) ;
#29560=DIRECTION ( 'NONE',  ( 0.000000000000000000, -1.000000000000000000, 0.000000000000000000 ) ) ;
#29566=CARTESIAN_POINT ( 'NONE',  ( 7.236395654485760609, 1.524999997268822183, -22.27133577429736633 ) ) ;
#29582=CARTESIAN_POINT ( 'NONE',  ( 14.47279130897151589, 12.82499999726882400, 19.92008829642072953 ) ) ;
#29633=CARTESIAN_POINT ( 'NONE',  ( 24.50000000000000000, 15.64999999453761248, 7.960532557706212486 ) ) ;
#29645=CARTESIAN_POINT ( 'NONE',  ( -15.14183272437242600, 11.29999999999999361, 20.84094480462497856 ) ) ;
#29649=CARTESIAN_POINT ( 'NONE',  ( -23.41746824999999887, 9.524999997268810858, -7.608796670333730638 ) ) ;
#29650=CARTESIAN_POINT ( 'NONE',  ( 7.570916362186213000, 4.399999999999987033, -23.30088464923126423 ) ) ;
#29653=CARTESIAN_POINT ( 'NONE',  ( 16.03387900638540842, 16.99999999999998224, -17.08446609624581569 ) ) ;
#29664=CARTESIAN_POINT ( 'NONE',  ( -24.49999999999965894, 16.89999999999998437, -7.960532557706680556 ) ) ;
#29683=CARTESIAN_POINT ( 'NONE',  ( -23.41746825000000598, 9.724999997268804819, 7.608796670333726198 ) ) ;
#29695=AXIS2_PLACEMENT_3D ( 'NONE', #27232, #32370, #6468 ) ;
#29707=CARTESIAN_POINT ( 'NONE',  ( 23.41746824999999887, 16.62499999726882294, 0.000000000000000000 ) ) ;
#29724=CYLINDRICAL_SURFACE ( 'NONE', #6991, 24.50000000000000000 ) ;
#29727=SURFACE_STYLE_USAGE ( .BOTH. , #1409 ) ;
#29734=CARTESIAN_POINT ( 'NONE',  ( 1.507698388325705758E-15, 9.624999997268808727, -24.62258325217400312 ) ) ;
#29751=CARTESIAN_POINT ( 'NONE',  ( 7.236395654485760609, 13.52499999726880553, -22.27133577429736633 ) ) ;
#29757=ORIENTED_EDGE ( 'NONE', *, *, #1373, .F. ) ;
#29783=CARTESIAN_POINT ( 'NONE',  ( 11.76128613161001368, 16.99999999999998579, 20.76574261957635059 ) ) ;
#29821=CARTESIAN_POINT ( 'NONE',  ( -15.14183272437241889, 10.70000000000001172, -20.84094480462497856 ) ) ;
#29825=CARTESIAN_POINT ( 'NONE',  ( 7.236395654485760609, 9.024999997268828622, -22.27133577429736633 ) ) ;
#29826=CARTESIAN_POINT ( 'NONE',  ( 19.82091636218621034, 3.549999994537617276, 14.40073868116559730 ) ) ;
#29829=EDGE_CURVE ( 'NONE', #22342, #16123, #13095, .T. ) ;
#29836=FACE_OUTER_BOUND ( 'NONE', #55, .T. ) ;
#29861=CARTESIAN_POINT ( 'NONE',  ( 7.236395654485755280, 14.22499999726881192, 22.27133577429736988 ) ) ;
#29872=DIRECTION ( 'NONE',  ( 0.000000000000000000, -1.000000000000000000, 0.000000000000000000 ) ) ;
#29886=CARTESIAN_POINT ( 'NONE',  ( -14.47279130897151767, 1.824999997268821783, -19.92008829642072598 ) ) ;
#29900=STYLED_ITEM ( 'NONE', ( #26997 ), #9785 ) ;
#29909=CARTESIAN_POINT ( 'NONE',  ( -7.236395654485757944, 5.724999997268803931, -22.27133577429736988 ) ) ;
#29925=CARTESIAN_POINT ( 'NONE',  ( 23.41746825000000243, 4.524999997268823293, 7.608796670333735079 ) ) ;
#29948=CARTESIAN_POINT ( 'NONE',  ( -7.570916362186215665, 7.149999994537637349, 23.30088464923126423 ) ) ;
#29955=CARTESIAN_POINT ( 'NONE',  ( 21.46812038053990079, 16.99999999999998934, 9.396489787187540799 ) ) ;
#29957=CARTESIAN_POINT ( 'NONE',  ( 15.14183272437242067, 1.700000000000004396, 20.84094480462498211 ) ) ;
#29977=EDGE_CURVE ( 'NONE', #23373, #27958, #8006, .T. ) ;
#29990=CARTESIAN_POINT ( 'NONE',  ( 24.50000000000000355, 13.89999999999999858, 7.960532557706212486 ) ) ;
#29994=CARTESIAN_POINT ( 'NONE',  ( 7.236395654485755280, 12.22499999726881015, 22.27133577429736988 ) ) ;
#30024=CARTESIAN_POINT ( 'NONE',  ( 1.555960095263670572E-15, 12.50000000000000355, -24.50000000000000000 ) ) ;
#30028=CARTESIAN_POINT ( 'NONE',  ( -23.41746824999999887, 9.624999997268817609, -2.867812753649727150E-15 ) ) ;
#30064=CARTESIAN_POINT ( 'NONE',  ( 0.000000000000000000, -20.99999999999998934, 0.000000000000000000 ) ) ;
#30071=CARTESIAN_POINT ( 'NONE',  ( -23.41746825000000598, 10.22499999726881903, 7.608796670333726198 ) ) ;
#30084=CARTESIAN_POINT ( 'NONE',  ( 18.94512977948576093, 2.824999997268817786, -13.76444248337722875 ) ) ;
#30110=CARTESIAN_POINT ( 'NONE',  ( 19.82091636218621389, 5.949999994537630066, -14.40073868116559197 ) ) ;
#30125=CARTESIAN_POINT ( 'NONE',  ( 1.507698388325705758E-15, 3.624999997268822938, -24.62258325217400312 ) ) ;
#30152=CARTESIAN_POINT ( 'NONE',  ( -4.732186688966233175E-15, 15.50000000000000533, 25.76082449383753925 ) ) ;
#30156=CARTESIAN_POINT ( 'NONE',  ( -7.236395654485757944, 13.22499999726881015, -22.27133577429736988 ) ) ;
#30160=EDGE_CURVE ( 'NONE', #11531, #33874, #18387, .T. ) ;
#30191=CARTESIAN_POINT ( 'NONE',  ( -4.523095164977116484E-15, 12.12499999726881406, 24.62258325217400312 ) ) ;
#30218=CARTESIAN_POINT ( 'NONE',  ( -23.41746824999999887, 2.024999997268815299, -7.608796670333730638 ) ) ;
#30234=CARTESIAN_POINT ( 'NONE',  ( 24.50000000000000000, 8.100000000000006750, -7.960532557706203605 ) ) ;
#30238=CARTESIAN_POINT ( 'NONE',  ( -4.523095164977116484E-15, 8.624999997268810503, 24.62258325217400312 ) ) ;
#30253=CARTESIAN_POINT ( 'NONE',  ( -23.41746824999999887, 5.624999997268814944, -2.867812753649727150E-15 ) ) ;
#30265=ADVANCED_FACE ( 'NONE', ( #33822 ), #8233, .T. ) ;
#30280=CARTESIAN_POINT ( 'NONE',  ( -15.14183272437241889, 6.449999994537612302, -20.84094480462497856 ) ) ;
#30289=CARTESIAN_POINT ( 'NONE',  ( 6.001560367445586717E-15, 1.500000000000005995, 24.50000000000000000 ) ) ;
#30308=CARTESIAN_POINT ( 'NONE',  ( -19.82091636218621034, 2.799999999999997158, -14.40073868116559552 ) ) ;
#30329=CARTESIAN_POINT ( 'NONE',  ( 23.41746824999999887, 16.52499999726882152, 7.608796670333735079 ) ) ;
#30333=CARTESIAN_POINT ( 'NONE',  ( -16.62822907945918871, 16.99999999999998934, -17.41050465759853694 ) ) ;
#30334=CARTESIAN_POINT ( 'NONE',  ( 23.95873412499999944, 1.437499995903229744, 0.000000000000000000 ) ) ;
#30363=CARTESIAN_POINT ( 'NONE',  ( 23.41746824999999887, 16.62499999726882294, 0.000000000000000000 ) ) ;
#30379=( GEOMETRIC_REPRESENTATION_CONTEXT ( 3 ) GLOBAL_UNCERTAINTY_ASSIGNED_CONTEXT ( ( #7438 ) ) GLOBAL_UNIT_ASSIGNED_CONTEXT ( ( #12529, #33973, #13555 ) ) REPRESENTATION_CONTEXT ( 'NONE', 'WORKASPACE' ) );
#30393=ORIENTED_EDGE ( 'NONE', *, *, #32495, .T. ) ;
#30413=CARTESIAN_POINT ( 'NONE',  ( -23.41746824999999887, 6.124999997268814944, -2.867812753649727150E-15 ) ) ;
#30426=CARTESIAN_POINT ( 'NONE',  ( 7.236395654485760609, 1.024999997268821739, -22.27133577429736633 ) ) ;
#30453=CARTESIAN_POINT ( 'NONE',  ( -7.570916362186210335, 6.349999994537613546, -23.30088464923126779 ) ) ;
#30461=CYLINDRICAL_SURFACE ( 'NONE', #25599, 24.50000000000000000 ) ;
#30478=CARTESIAN_POINT ( 'NONE',  ( -19.82091636218621389, 8.949999994537632730, 14.40073868116558842 ) ) ;
#30493=CARTESIAN_POINT ( 'NONE',  ( -19.82091636218621389, 15.19999999999999218, 14.40073868116558842 ) ) ;
#30498=CARTESIAN_POINT ( 'NONE',  ( 0.000000000000000000, 16.99999999999998579, -24.50000000000000000 ) ) ;
#30536=CARTESIAN_POINT ( 'NONE',  ( -7.236395654485763274, 18.02499999726880731, 22.27133577429736633 ) ) ;
#30561=CARTESIAN_POINT ( 'NONE',  ( -18.94512977948576093, 10.32499999726882400, 13.76444248337722698 ) ) ;
#30579=DIRECTION ( 'NONE',  ( 0.8660254037844399289, -0.4999999999999977240, 0.000000000000000000 ) ) ;
#30586=CARTESIAN_POINT ( 'NONE',  ( -7.236395654485763274, 10.52499999726880198, 22.27133577429736633 ) ) ;
#30600=CARTESIAN_POINT ( 'NONE',  ( 23.41746824999999887, 2.624999997268812280, 0.000000000000000000 ) ) ;
#30607=EDGE_LOOP ( 'NONE', ( #32459, #2900, #22460, #6539 ) ) ;
#30623=CARTESIAN_POINT ( 'NONE',  ( -4.732186688966233175E-15, 15.24999999453762811, 25.76082449383753925 ) ) ;
#30632=ADVANCED_FACE ( 'NONE', ( #29836 ), #505, .T. ) ;
#30650=CARTESIAN_POINT ( 'NONE',  ( -3.880418787951136483, 8.301254276084460315, -24.50000000000000000 ) ) ;
#30656=CARTESIAN_POINT ( 'NONE',  ( -7.570916362186210335, 4.599999999999992539, -23.30088464923126779 ) ) ;
#30670=CARTESIAN_POINT ( 'NONE',  ( 8.998893468610761559, 16.99999999999998579, -21.61938333025141290 ) ) ;
#30674=CARTESIAN_POINT ( 'NONE',  ( -24.11383999230005415, 17.00000000000000355, -3.930170939105292138 ) ) ;
#30703=CARTESIAN_POINT ( 'NONE',  ( 1.555960095263670572E-15, 16.24999999453762101, -24.50000000000000000 ) ) ;
#30708=CARTESIAN_POINT ( 'NONE',  ( -7.236395654485763274, 16.02499999726880731, 22.27133577429736633 ) ) ;
#30709=( BOUNDED_CURVE ( )  B_SPLINE_CURVE ( 2, ( #14027, #963, #3888, #11444, #14360, #21920, #469, #6296, #10952, #16772, #8363, #28249, #4226 ),
 .UNSPECIFIED., .F., .T. ) 
 B_SPLINE_CURVE_WITH_KNOTS ( ( 3, 2, 2, 2, 2, 2, 3 ),
 ( 0.4722222222222222654, 0.4777777777777778012, 0.4888888888888888729, 0.5000000000000000000, 0.5111111111111110716, 0.5222222222222222543, 0.5277777777777777901 ),
 .UNSPECIFIED. ) 
 CURVE ( )  GEOMETRIC_REPRESENTATION_ITEM ( )  RATIONAL_B_SPLINE_CURVE ( ( 0.9755282581475767101, 0.9755282581475768211, 1.000000000000000000, 0.9510565162951535312, 1.000000000000000000, 0.9510565162951535312, 1.000000000000000000, 0.9510565162951535312, 1.000000000000000000, 0.9510565162951535312, 1.000000000000000000, 0.9755282581475768211, 0.9755282581475768211 ) ) 
 REPRESENTATION_ITEM ( '' )  );
#30715=ORIENTED_EDGE ( 'NONE', *, *, #549, .F. ) ;
#30724=CARTESIAN_POINT ( 'NONE',  ( 24.50000000000000000, 6.100000000000011191, -7.960532557706203605 ) ) ;
#30734=CARTESIAN_POINT ( 'NONE',  ( 14.47279130897151767, 10.82499999726882756, 19.92008829642072953 ) ) ;
#30760=CARTESIAN_POINT ( 'NONE',  ( 7.236395654485755280, 12.72499999726881015, 22.27133577429736988 ) ) ;
#30761=CARTESIAN_POINT ( 'NONE',  ( 7.236395654485755280, 4.224999997268802154, 22.27133577429736988 ) ) ;
#30775=CARTESIAN_POINT ( 'NONE',  ( 23.41746825000000243, 8.724999997268806595, -7.608796670333727974 ) ) ;
#30777=ORIENTED_EDGE ( 'NONE', *, *, #32304, .F. ) ;
#30798=CARTESIAN_POINT ( 'NONE',  ( -24.50000000000001066, 14.84999999453764019, 7.960532557706201828 ) ) ;
#30812=CARTESIAN_POINT ( 'NONE',  ( 18.94512977948576093, 3.324999997268818230, -13.76444248337722875 ) ) ;
#30821=ORIENTED_EDGE ( 'NONE', *, *, #16507, .T. ) ;
#30824=CARTESIAN_POINT ( 'NONE',  ( 19.82091636218621389, 10.20000000000001528, -14.40073868116559197 ) ) ;
#30826=CARTESIAN_POINT ( 'NONE',  ( -7.570916362186215665, 9.149999994537639125, 23.30088464923126423 ) ) ;
#30844=CARTESIAN_POINT ( 'NONE',  ( -7.570916362186210335, 16.60000000000000497, -23.30088464923126779 ) ) ;
#30849=CARTESIAN_POINT ( 'NONE',  ( -14.47279130897151767, 15.32499999726880269, -19.92008829642072598 ) ) ;
#30852=CARTESIAN_POINT ( 'NONE',  ( 23.23218422517957293, 16.99999999999997868, 3.037944173731645936 ) ) ;
#30855=DIRECTION ( 'NONE',  ( 0.000000000000000000, 0.000000000000000000, -1.000000000000000000 ) ) ;
#30856=CARTESIAN_POINT ( 'NONE',  ( 0.000000000000000000, -20.99999999999998934, 0.000000000000000000 ) ) ;
#30883=CARTESIAN_POINT ( 'NONE',  ( 15.14183272437242245, 0.2999999999999904965, -20.84094480462497856 ) ) ;
#30910=CARTESIAN_POINT ( 'NONE',  ( -7.236395654485757944, 7.724999997268805707, -22.27133577429736988 ) ) ;
#30911=ORIENTED_EDGE ( 'NONE', *, *, #3287, .F. ) ;
#30936=CARTESIAN_POINT ( 'NONE',  ( -14.47279130897152122, 12.42499999726880766, 19.92008829642072243 ) ) ;
#30937=CARTESIAN_POINT ( 'NONE',  ( -23.41746825000000243, 1.724999997268824581, 7.608796670333725309 ) ) ;
#30949=CARTESIAN_POINT ( 'NONE',  ( -18.94512977948576093, 11.82499999726882578, 13.76444248337722698 ) ) ;
#30973=CARTESIAN_POINT ( 'NONE',  ( 15.14183272437241889, 11.44999999453763095, 20.84094480462498211 ) ) ;
#30988=CARTESIAN_POINT ( 'NONE',  ( 18.94512977948576093, 11.32499999726882578, -13.76444248337722875 ) ) ;
#30991=AXIS2_PLACEMENT_3D ( 'NONE', #25404, #28149, #1882 ) ;
#30997=ORIENTED_EDGE ( 'NONE', *, *, #22429, .F. ) ;
#31028=CARTESIAN_POINT ( 'NONE',  ( 3.445340210940985210E-14, 5.499999999999997335, 24.50000000000000000 ) ) ;
#31048=CARTESIAN_POINT ( 'NONE',  ( 0.000000000000000000, 16.99999999999998579, 0.000000000000000000 ) ) ;
#31059=CARTESIAN_POINT ( 'NONE',  ( 24.50000000000000355, 1.899999999999998135, 7.960532557706212486 ) ) ;
#31061=CARTESIAN_POINT ( 'NONE',  ( 1.836970198721029589E-15, 16.99999999999998579, 15.00000000000000000 ) ) ;
#31069=DIRECTION ( 'NONE',  ( 0.000000000000000000, -1.000000000000000000, 0.000000000000000000 ) ) ;
#31070=CARTESIAN_POINT ( 'NONE',  ( 24.50000000000000000, 6.000000000000005329, 0.000000000000000000 ) ) ;
#31077=CARTESIAN_POINT ( 'NONE',  ( 19.82091636218621389, 0.2000000000000057288, -14.40073868116559197 ) ) ;
#31078=ADVANCED_FACE ( 'NONE', ( #10443 ), #15428, .T. ) ;
#31082=CARTESIAN_POINT ( 'NONE',  ( 14.47279130897151767, 4.824999997268814234, 19.92008829642072953 ) ) ;
#31098=CARTESIAN_POINT ( 'NONE',  ( 14.47279130897151767, 0.9249999972688209837, -19.92008829642072598 ) ) ;
#31108=CARTESIAN_POINT ( 'NONE',  ( 1.507698388325705758E-15, 11.62499999726880340, -24.62258325217400312 ) ) ;
#31109=CARTESIAN_POINT ( 'NONE',  ( -23.41746824999999887, 1.524999997268801755, -7.608796670333730638 ) ) ;
#31122=CARTESIAN_POINT ( 'NONE',  ( -18.94512977948575738, 7.424999997268811214, -13.76444248337723231 ) ) ;
#31134=EDGE_LOOP ( 'NONE', ( #24234, #25254, #28544, #3898 ) ) ;
#31148=CARTESIAN_POINT ( 'NONE',  ( -7.570916362186215665, 13.14999999453761426, 23.30088464923126423 ) ) ;
#31161=CARTESIAN_POINT ( 'NONE',  ( -23.41746824999999887, 10.12499999726881938, -2.867812753649727150E-15 ) ) ;
#31167=ORIENTED_EDGE ( 'NONE', *, *, #5376, .F. ) ;
#31174=EDGE_CURVE ( 'NONE', #17247, #33874, #13992, .T. ) ;
#31186=EDGE_CURVE ( 'NONE', #14369, #6559, #17832, .T. ) ;
#31227=CARTESIAN_POINT ( 'NONE',  ( -19.82091636218621389, 3.200000000000008171, 14.40073868116558842 ) ) ;
#31250=CARTESIAN_POINT ( 'NONE',  ( -23.41746824999999887, 10.12499999726881938, -2.867812753649727150E-15 ) ) ;
#31266=CARTESIAN_POINT ( 'NONE',  ( -18.94512977948575738, 5.424999997268809437, -13.76444248337723231 ) ) ;
#31277=CARTESIAN_POINT ( 'NONE',  ( -18.94512977948575738, 15.92499999726881832, -13.76444248337723231 ) ) ;
#31288=CARTESIAN_POINT ( 'NONE',  ( -4.523095164977116484E-15, 6.124999997268802510, 24.62258325217400312 ) ) ;
#31315=CARTESIAN_POINT ( 'NONE',  ( -24.50000000000000355, 14.64999999453761603, -7.960532557706207157 ) ) ;
#31331=CARTESIAN_POINT ( 'NONE',  ( 1.507698388325705758E-15, 7.624999997268814056, -24.62258325217400312 ) ) ;
#31347=CARTESIAN_POINT ( 'NONE',  ( -3.880418787951146697, 4.551254281546843750, -24.49999999999999645 ) ) ;
#31377=ORIENTED_EDGE ( 'NONE', *, *, #33041, .F. ) ;
#31397=CARTESIAN_POINT ( 'NONE',  ( 24.50000000000000000, 4.000000000000003553, 0.000000000000000000 ) ) ;
#31399=CARTESIAN_POINT ( 'NONE',  ( -24.50000000000000000, 2.749999994537621895, -3.000384657911015469E-15 ) ) ;
#31421=CARTESIAN_POINT ( 'NONE',  ( 23.41746824999999887, 13.22499999726881192, -7.608796670333727974 ) ) ;
#31438=CARTESIAN_POINT ( 'NONE',  ( -23.41746825000000243, 3.524999997268826402, -7.608796670333730638 ) ) ;
#31460=CARTESIAN_POINT ( 'NONE',  ( 23.41746825000000243, 10.72499999726880127, -7.608796670333727974 ) ) ;
#31461=CARTESIAN_POINT ( 'NONE',  ( 24.50000000000000000, 14.09999999999999076, -7.960532557706203605 ) ) ;
#31487=CARTESIAN_POINT ( 'NONE',  ( -7.570916362186210335, 18.34999999453762598, -23.30088464923126779 ) ) ;
#31494=CARTESIAN_POINT ( 'NONE',  ( -24.50000000000000000, 7.000000000000006217, -3.000384657911015469E-15 ) ) ;
#31501=CARTESIAN_POINT ( 'NONE',  ( -7.236395654485763274, 8.524999997268828622, 22.27133577429736633 ) ) ;
#31539=CARTESIAN_POINT ( 'NONE',  ( -19.82091636218621389, 12.94999999453763628, 14.40073868116558842 ) ) ;
#31560=CARTESIAN_POINT ( 'NONE',  ( -15.14183272437242600, 3.300000000000012257, 20.84094480462497856 ) ) ;
#31562=CARTESIAN_POINT ( 'NONE',  ( -24.50000000000000355, 2.649999994537616477, -7.960532557706207157 ) ) ;
#31583=CARTESIAN_POINT ( 'NONE',  ( 1.507698388325705758E-15, 15.62499999726882116, -24.62258325217400312 ) ) ;
#31601=CARTESIAN_POINT ( 'NONE',  ( 23.41746824999999887, 6.624999997268815832, 0.000000000000000000 ) ) ;
#31623=CARTESIAN_POINT ( 'NONE',  ( 7.236395654485755280, 18.22499999726881370, 22.27133577429736988 ) ) ;
#31649=CARTESIAN_POINT ( 'NONE',  ( 23.41746825000000243, 3.024999997268812635, 7.608796670333735079 ) ) ;
#31657=CARTESIAN_POINT ( 'NONE',  ( -19.82091636218621389, 7.200000000000011724, 14.40073868116558842 ) ) ;
#31664=CARTESIAN_POINT ( 'NONE',  ( -4.523095164977116484E-15, 6.624999997268815832, 24.62258325217400312 ) ) ;
#31674=ORIENTED_EDGE ( 'NONE', *, *, #12497, .F. ) ;
#31693=EDGE_CURVE ( 'NONE', #14415, #13367, #11159, .T. ) ;
#31713=EDGE_LOOP ( 'NONE', ( #29757, #2298, #3482, #13234 ) ) ;
#31729=CARTESIAN_POINT ( 'NONE',  ( -15.14183272437242600, 7.300000000000001599, 20.84094480462497856 ) ) ;
#31734=CARTESIAN_POINT ( 'NONE',  ( 23.41746824999999887, 4.624999997268814056, 0.000000000000000000 ) ) ;
#31735=CARTESIAN_POINT ( 'NONE',  ( 3.880418787951132042, 4.198745712990783474, -24.50000000000000355 ) ) ;
#31752=CARTESIAN_POINT ( 'NONE',  ( 23.41746824999999887, 13.12499999726882116, 0.000000000000000000 ) ) ;
#31767=CARTESIAN_POINT ( 'NONE',  ( -23.41746825000000598, 7.724999997268809260, 7.608796670333726198 ) ) ;
#31789=CARTESIAN_POINT ( 'NONE',  ( 23.41746825000000243, 14.72499999726881903, -7.608796670333727974 ) ) ;
#31792=VERTEX_POINT ( 'NONE', #29085 ) ;
#31806=CARTESIAN_POINT ( 'NONE',  ( -7.570916362186215665, 7.149999994537637349, 23.30088464923126423 ) ) ;
#31816=CARTESIAN_POINT ( 'NONE',  ( 15.14183272437242245, 18.04999999453762172, -20.84094480462497856 ) ) ;
#31819=( BOUNDED_SURFACE ( )  B_SPLINE_SURFACE ( 1, 2, ( 
 ( #32971, #4501, #2271, #31098, #25446, #15498, #19957, #12399, #2098, #6903, #28186, #17384, #25618, #13426, #26797, #28862, #5192, #10346, #2785, #29362, #31935, #18247, #18417, #20822, #13251, #3127, #5359, #8428, #20988, #31438, #21159, #28694, #21326, #15676, #26124, #29026, #23389, #22, #8260, #16177, #13084, #18752, #3291, #23724, #26464, #26633, #15839, #13599, #31266, #23894, #33851, #26296, #2621, #7761, #191, #5863, #18917, #23558, #10678, #10510, #31601, #24065, #8099, #16341, #7930, #18586, #5529, #16009, #2956, #365, #10851, #31767, #29194, #5700, #531, #11018, #21488, #24716, #6693, #9099, #14095, #14428, #11183, #3621, #6533, #11843, #22322, #32268, #3453, #3788, #30028, #29683, #27635, #21654, #32767, #1193, #27296, #9261, #27463, #3953, #19080, #1366, #8761, #32099, #6023, #6188, #21985, #24389, #32599, #17006, #19580, #27127, #24883, #19745, #8596, #30191, #697, #24551, #863, #17177, #19244, #29520, #1023, #13756, #11505, #16501, #16670, #24227, #32433, #11674, #8931, #26954, #19412, #13925, #11344, #21820, #29861, #6361, #22157, #16840, #14258, #33458, #22653, #1536, #33286, #25742, #17863, #14765, #9783, #12012, #20263, #33105, #14937, #9610, #30708, #17515, #12532, #12357, #7032, #2224, #30363, #2056, #9429, #10133, #9957, #20091, #22481, #7203, #12701, #28314, #25230, #17687, #32930, #28147, #30536, #25402, #27976, #4633, #4461, #23001, #22826 ),
 ( #4123, #1704, #20433, #30883, #27806, #7379, #7552, #1880, #15112, #4802, #25576, #15282, #19914, #23172, #18036, #33634, #6864, #25055, #20615, #31059, #14598, #17343, #4290, #12183, #18376, #8220, #23516, #3088, #26085, #2581, #26255, #15633, #31227, #31560, #13560, #18543, #21117, #24022, #10305, #10469, #31397, #5488, #21449, #23856, #28821, #29150, #25911, #5319, #21289, #26592, #492, #13045, #18207, #28989, #10809, #20948, #8388, #2405, #10975, #15967, #8058, #31892, #18714, #5656, #33812, #16138, #33976, #12873, #20783, #7887, #2743, #5146, #13384, #31729, #322, #15799, #28482, #4978, #23350, #15456, #7720, #13207, #23683, #28650, #149, #10638, #26423, #2917, #6147, #5824, #826, #22118, #3582, #16801, #8723, #16302, #3415, #26759, #1324, #24845, #27425, #8890, #11471, #3916, #658, #11307, #21785, #29821, #11806, #14223, #19207, #19542, #3251, #29645, #11635, #16967, #14388, #13889, #8561, #19375, #1153, #32233, #32729, #13721, #22284, #6325, #32396, #18873, #32562, #9061, #24186, #6494, #24356, #11146, #21616, #16632, #27088, #29483, #3749, #29990, #24679, #14054, #29322, #32061, #19045, #5987, #16464, #24516, #26919, #986, #21945, #27258, #30493, #20392, #6994, #30152, #25187, #12491, #27937, #7162, #33065, #6656, #27765, #17139, #25703, #15241, #30844, #1497, #17645, #14556, #2184, #4593, #4251, #27592, #4421, #7335, #22960, #19872, #14896, #4083, #25360 ) ),
 .UNSPECIFIED., .F., .F., .T. ) 
 B_SPLINE_SURFACE_WITH_KNOTS ( ( 2, 2 ),
 ( 3, 2, 2, 2, 2, 2, 2, 2, 2, 2, 2, 2, 2, 2, 2, 2, 2, 2, 2, 2, 2, 2, 2, 2, 2, 2, 2, 2, 2, 2, 2, 2, 2, 2, 2, 2, 2, 2, 2, 2, 2, 2, 2, 2, 2, 2, 2, 2, 2, 2, 2, 2, 2, 2, 2, 2, 2, 2, 2, 2, 2, 2, 2, 2, 2, 2, 2, 2, 2, 2, 2, 2, 2, 2, 2, 2, 2, 2, 2, 2, 2, 2, 2, 2, 2, 2, 2, 2, 2, 2, 3 ),
 ( 0.000000000000000000, 1.000000000000000000 ),
 ( 0.000000000000000000, 0.01111111111111111154, 0.02222222222222222307, 0.03333333333333333287, 0.04444444444444444614, 0.05555555555555555247, 0.06666666666666666574, 0.07777777777777777901, 0.08888888888888889228, 0.1000000000000000056, 0.1111111111111111049, 0.1222222222222222182, 0.1333333333333333315, 0.1444444444444444309, 0.1555555555555555580, 0.1666666666666666574, 0.1777777777777777846, 0.1888888888888888840, 0.2000000000000000111, 0.2111111111111111105, 0.2222222222222222099, 0.2333333333333333370, 0.2444444444444444364, 0.2555555555555555358, 0.2666666666666666630, 0.2777777777777777901, 0.2888888888888888618, 0.2999999999999999889, 0.3111111111111111160, 0.3222222222222222432, 0.3333333333333333148, 0.3444444444444444420, 0.3555555555555555691, 0.3666666666666666408, 0.3777777777777777679, 0.3888888888888888951, 0.4000000000000000222, 0.4111111111111110938, 0.4222222222222222210, 0.4333333333333333481, 0.4444444444444444198, 0.4555555555555555469, 0.4666666666666666741, 0.4777777777777778012, 0.4888888888888888729, 0.5000000000000000000, 0.5111111111111110716, 0.5222222222222222543, 0.5333333333333333259, 0.5444444444444443976, 0.5555555555555555802, 0.5666666666666666519, 0.5777777777777777235, 0.5888888888888889062, 0.5999999999999999778, 0.6111111111111111605, 0.6222222222222222321, 0.6333333333333333037, 0.6444444444444444864, 0.6555555555555555580, 0.6666666666666666297, 0.6777777777777778123, 0.6888888888888888840, 0.6999999999999999556, 0.7111111111111111382, 0.7222222222222222099, 0.7333333333333332815, 0.7444444444444444642, 0.7555555555555555358, 0.7666666666666667185, 0.7777777777777777901, 0.7888888888888888618, 0.8000000000000000444, 0.8111111111111111160, 0.8222222222222221877, 0.8333333333333333703, 0.8444444444444444420, 0.8555555555555555136, 0.8666666666666666963, 0.8777777777777777679, 0.8888888888888888395, 0.9000000000000000222, 0.9111111111111110938, 0.9222222222222222765, 0.9333333333333333481, 0.9444444444444444198, 0.9555555555555556024, 0.9666666666666666741, 0.9777777777777777457, 0.9888888888888889284, 1.000000000000000000 ),
 .UNSPECIFIED. ) 
 GEOMETRIC_REPRESENTATION_ITEM ( )  RATIONAL_B_SPLINE_SURFACE ( (
 ( 1.000000000000000000, 0.9510565162951535312, 1.000000000000000000, 0.9510565162951535312, 1.000000000000000000, 0.9510565162951535312, 1.000000000000000000, 0.9510565162951535312, 1.000000000000000000, 0.9510565162951535312, 1.000000000000000000, 0.9510565162951535312, 1.000000000000000000, 0.9510565162951535312, 1.000000000000000000, 0.9510565162951535312, 1.000000000000000000, 0.9510565162951535312, 1.000000000000000000, 0.9510565162951535312, 1.000000000000000000, 0.9510565162951535312, 1.000000000000000000, 0.9510565162951535312, 1.000000000000000000, 0.9510565162951535312, 1.000000000000000000, 0.9510565162951535312, 1.000000000000000000, 0.9510565162951535312, 1.000000000000000000, 0.9510565162951535312, 1.000000000000000000, 0.9510565162951535312, 1.000000000000000000, 0.9510565162951535312, 1.000000000000000000, 0.9510565162951535312, 1.000000000000000000, 0.9510565162951535312, 1.000000000000000000, 0.9510565162951535312, 1.000000000000000000, 0.9510565162951535312, 1.000000000000000000, 0.9510565162951535312, 1.000000000000000000, 0.9510565162951535312, 1.000000000000000000, 0.9510565162951535312, 1.000000000000000000, 0.9510565162951535312, 1.000000000000000000, 0.9510565162951535312, 1.000000000000000000, 0.9510565162951535312, 1.000000000000000000, 0.9510565162951535312, 1.000000000000000000, 0.9510565162951535312, 1.000000000000000000, 0.9510565162951535312, 1.000000000000000000, 0.9510565162951535312, 1.000000000000000000, 0.9510565162951535312, 1.000000000000000000, 0.9510565162951535312, 1.000000000000000000, 0.9510565162951535312, 1.000000000000000000, 0.9510565162951535312, 1.000000000000000000, 0.9510565162951535312, 1.000000000000000000, 0.9510565162951535312, 1.000000000000000000, 0.9510565162951535312, 1.000000000000000000, 0.9510565162951535312, 1.000000000000000000, 0.9510565162951535312, 1.000000000000000000, 0.9510565162951535312, 1.000000000000000000, 0.9510565162951535312, 1.000000000000000000, 0.9510565162951535312, 1.000000000000000000, 0.9510565162951535312, 1.000000000000000000, 0.9510565162951535312, 1.000000000000000000, 0.9510565162951535312, 1.000000000000000000, 0.9510565162951535312, 1.000000000000000000, 0.9510565162951535312, 1.000000000000000000, 0.9510565162951535312, 1.000000000000000000, 0.9510565162951535312, 1.000000000000000000, 0.9510565162951535312, 1.000000000000000000, 0.9510565162951535312, 1.000000000000000000, 0.9510565162951535312, 1.000000000000000000, 0.9510565162951535312, 1.000000000000000000, 0.9510565162951535312, 1.000000000000000000, 0.9510565162951535312, 1.000000000000000000, 0.9510565162951535312, 1.000000000000000000, 0.9510565162951535312, 1.000000000000000000, 0.9510565162951535312, 1.000000000000000000, 0.9510565162951535312, 1.000000000000000000, 0.9510565162951535312, 1.000000000000000000, 0.9510565162951535312, 1.000000000000000000, 0.9510565162951535312, 1.000000000000000000, 0.9510565162951535312, 1.000000000000000000, 0.9510565162951535312, 1.000000000000000000, 0.9510565162951535312, 1.000000000000000000, 0.9510565162951535312, 1.000000000000000000, 0.9510565162951535312, 1.000000000000000000, 0.9510565162951535312, 1.000000000000000000, 0.9510565162951535312, 1.000000000000000000, 0.9510565162951535312, 1.000000000000000000, 0.9510565162951535312, 1.000000000000000000, 0.9510565162951535312, 1.000000000000000000, 0.9510565162951535312, 1.000000000000000000, 0.9510565162951535312, 1.000000000000000000, 0.9510565162951535312, 1.000000000000000000, 0.9510565162951535312, 1.000000000000000000, 0.9510565162951535312, 1.000000000000000000, 0.9510565162951535312, 1.000000000000000000, 0.9510565162951535312, 1.000000000000000000, 0.9510565162951535312, 1.000000000000000000, 0.9510565162951535312, 1.000000000000000000, 0.9510565162951535312, 1.000000000000000000, 0.9510565162951535312, 1.000000000000000000, 0.9510565162951535312, 1.000000000000000000, 0.9510565162951535312, 1.000000000000000000, 0.9510565162951535312, 1.000000000000000000, 0.9510565162951535312, 1.000000000000000000, 0.9510565162951535312, 1.000000000000000000),
 ( 1.000000000000000000, 0.9510565162951535312, 1.000000000000000000, 0.9510565162951535312, 1.000000000000000000, 0.9510565162951535312, 1.000000000000000000, 0.9510565162951535312, 1.000000000000000000, 0.9510565162951535312, 1.000000000000000000, 0.9510565162951535312, 1.000000000000000000, 0.9510565162951535312, 1.000000000000000000, 0.9510565162951535312, 1.000000000000000000, 0.9510565162951535312, 1.000000000000000000, 0.9510565162951535312, 1.000000000000000000, 0.9510565162951535312, 1.000000000000000000, 0.9510565162951535312, 1.000000000000000000, 0.9510565162951535312, 1.000000000000000000, 0.9510565162951535312, 1.000000000000000000, 0.9510565162951535312, 1.000000000000000000, 0.9510565162951535312, 1.000000000000000000, 0.9510565162951535312, 1.000000000000000000, 0.9510565162951535312, 1.000000000000000000, 0.9510565162951535312, 1.000000000000000000, 0.9510565162951535312, 1.000000000000000000, 0.9510565162951535312, 1.000000000000000000, 0.9510565162951535312, 1.000000000000000000, 0.9510565162951535312, 1.000000000000000000, 0.9510565162951535312, 1.000000000000000000, 0.9510565162951535312, 1.000000000000000000, 0.9510565162951535312, 1.000000000000000000, 0.9510565162951535312, 1.000000000000000000, 0.9510565162951535312, 1.000000000000000000, 0.9510565162951535312, 1.000000000000000000, 0.9510565162951535312, 1.000000000000000000, 0.9510565162951535312, 1.000000000000000000, 0.9510565162951535312, 1.000000000000000000, 0.9510565162951535312, 1.000000000000000000, 0.9510565162951535312, 1.000000000000000000, 0.9510565162951535312, 1.000000000000000000, 0.9510565162951535312, 1.000000000000000000, 0.9510565162951535312, 1.000000000000000000, 0.9510565162951535312, 1.000000000000000000, 0.9510565162951535312, 1.000000000000000000, 0.9510565162951535312, 1.000000000000000000, 0.9510565162951535312, 1.000000000000000000, 0.9510565162951535312, 1.000000000000000000, 0.9510565162951535312, 1.000000000000000000, 0.9510565162951535312, 1.000000000000000000, 0.9510565162951535312, 1.000000000000000000, 0.9510565162951535312, 1.000000000000000000, 0.9510565162951535312, 1.000000000000000000, 0.9510565162951535312, 1.000000000000000000, 0.9510565162951535312, 1.000000000000000000, 0.9510565162951535312, 1.000000000000000000, 0.9510565162951535312, 1.000000000000000000, 0.9510565162951535312, 1.000000000000000000, 0.9510565162951535312, 1.000000000000000000, 0.9510565162951535312, 1.000000000000000000, 0.9510565162951535312, 1.000000000000000000, 0.9510565162951535312, 1.000000000000000000, 0.9510565162951535312, 1.000000000000000000, 0.9510565162951535312, 1.000000000000000000, 0.9510565162951535312, 1.000000000000000000, 0.9510565162951535312, 1.000000000000000000, 0.9510565162951535312, 1.000000000000000000, 0.9510565162951535312, 1.000000000000000000, 0.9510565162951535312, 1.000000000000000000, 0.9510565162951535312, 1.000000000000000000, 0.9510565162951535312, 1.000000000000000000, 0.9510565162951535312, 1.000000000000000000, 0.9510565162951535312, 1.000000000000000000, 0.9510565162951535312, 1.000000000000000000, 0.9510565162951535312, 1.000000000000000000, 0.9510565162951535312, 1.000000000000000000, 0.9510565162951535312, 1.000000000000000000, 0.9510565162951535312, 1.000000000000000000, 0.9510565162951535312, 1.000000000000000000, 0.9510565162951535312, 1.000000000000000000, 0.9510565162951535312, 1.000000000000000000, 0.9510565162951535312, 1.000000000000000000, 0.9510565162951535312, 1.000000000000000000, 0.9510565162951535312, 1.000000000000000000, 0.9510565162951535312, 1.000000000000000000, 0.9510565162951535312, 1.000000000000000000, 0.9510565162951535312, 1.000000000000000000, 0.9510565162951535312, 1.000000000000000000, 0.9510565162951535312, 1.000000000000000000, 0.9510565162951535312, 1.000000000000000000, 0.9510565162951535312, 1.000000000000000000, 0.9510565162951535312, 1.000000000000000000, 0.9510565162951535312, 1.000000000000000000, 0.9510565162951535312, 1.000000000000000000, 0.9510565162951535312, 1.000000000000000000, 0.9510565162951535312, 1.000000000000000000) ) ) 
 REPRESENTATION_ITEM ( '' )  SURFACE ( )  );
#31830=CARTESIAN_POINT ( 'NONE',  ( -7.236395654485757944, 17.72499999726881370, -22.27133577429736988 ) ) ;
#31870=CARTESIAN_POINT ( 'NONE',  ( -15.14183272437242067, 12.70000000000000639, -20.84094480462497856 ) ) ;
#31876=EDGE_CURVE ( 'NONE', #24787, #28001, #15094, .T. ) ;
#31892=CARTESIAN_POINT ( 'NONE',  ( 24.50000000000000355, 6.100000000000010303, -7.960532557706203605 ) ) ;
#31897=CARTESIAN_POINT ( 'NONE',  ( -14.47279130897151767, 1.324999997268808238, -19.92008829642072598 ) ) ;
#31898=CARTESIAN_POINT ( 'NONE',  ( 7.570916362186213000, 4.149999994537633796, -23.30088464923126423 ) ) ;
#31901=CARTESIAN_POINT ( 'NONE',  ( 13.67209884950243470, 16.99999999999998934, -19.02727893622179423 ) ) ;
#31906=DIRECTION ( 'NONE',  ( 0.000000000000000000, -1.000000000000000000, 0.000000000000000000 ) ) ;
#31915=AXIS2_PLACEMENT_3D ( 'NONE', #12564, #4837, #25610 ) ;
#31919=CARTESIAN_POINT ( 'NONE',  ( 1.507698388325705758E-15, 13.62499999726882649, -24.62258325217400312 ) ) ;
#31920=ORIENTED_EDGE ( 'NONE', *, *, #5240, .T. ) ;
#31935=CARTESIAN_POINT ( 'NONE',  ( 23.41746824999999887, 2.624999997268812280, 0.000000000000000000 ) ) ;
#31943=ORIENTED_EDGE ( 'NONE', *, *, #18402, .T. ) ;
#31957=CARTESIAN_POINT ( 'NONE',  ( 7.236395654485755280, 16.22499999726881370, 22.27133577429736988 ) ) ;
#31959=ORIENTED_EDGE ( 'NONE', *, *, #9685, .F. ) ;
#31976=DIRECTION ( 'NONE',  ( 0.000000000000000000, -1.000000000000000000, 0.000000000000000000 ) ) ;
#31982=CARTESIAN_POINT ( 'NONE',  ( -19.82091636218621034, 18.54999999453762882, -14.40073868116559552 ) ) ;
#31997=CARTESIAN_POINT ( 'NONE',  ( -23.41746824999999887, 18.12499999726882649, -2.867812753649727150E-15 ) ) ;
#32023=CARTESIAN_POINT ( 'NONE',  ( -3.880418787951104953, 11.44874571845314293, 24.50000000000000711 ) ) ;
#32030=CARTESIAN_POINT ( 'NONE',  ( -0.4126531432213792483, 16.99999999999998579, 24.09281253189301353 ) ) ;
#32047=CARTESIAN_POINT ( 'NONE',  ( 15.14183272437242067, 15.44999999453762207, 20.84094480462498211 ) ) ;
#32061=CARTESIAN_POINT ( 'NONE',  ( 15.14183272437242245, 14.30000000000001315, -20.84094480462497856 ) ) ;
#32064=CARTESIAN_POINT ( 'NONE',  ( 1.507698388325705758E-15, 9.124999997268822938, -24.62258325217400312 ) ) ;
#32065=CARTESIAN_POINT ( 'NONE',  ( -4.223320258572819786E-15, 9.499999999999992895, 24.50000000000000000 ) ) ;
#32086=CARTESIAN_POINT ( 'NONE',  ( -7.236395654485757944, 11.72499999726880837, -22.27133577429736988 ) ) ;
#32094=PRODUCT ( 'connector', 'connector', '', ( #280 ) ) ;
#32099=CARTESIAN_POINT ( 'NONE',  ( 14.47279130897151767, 10.92499999726882365, -19.92008829642072598 ) ) ;
#32107=CARTESIAN_POINT ( 'NONE',  ( -4.523095164977116484E-15, 18.62499999726881583, 24.62258325217400312 ) ) ;
#32109=ADVANCED_FACE ( 'NONE', ( #5165 ), #26272, .F. ) ;
#32122=( BOUNDED_CURVE ( )  B_SPLINE_CURVE ( 2, ( #32301, #10884, #26989, #8293, #11536, #6053, #21359, #5897, #3488, #16537, #26666, #8463, #18622 ),
 .UNSPECIFIED., .F., .T. ) 
 B_SPLINE_CURVE_WITH_KNOTS ( ( 3, 2, 2, 2, 2, 2, 3 ),
 ( 0.02777777777777777971, 0.03333333333333333287, 0.04444444444444444614, 0.05555555555555555247, 0.06666666666666667962, 0.07777777777777777901, 0.08333333333333334259 ),
 .UNSPECIFIED. ) 
 CURVE ( )  GEOMETRIC_REPRESENTATION_ITEM ( )  RATIONAL_B_SPLINE_CURVE ( ( 0.9755282581475768211, 0.9755282581475768211, 1.000000000000000000, 0.9510565162951535312, 1.000000000000000000, 0.9510565162951535312, 1.000000000000000000, 0.9510565162951535312, 1.000000000000000000, 0.9510565162951535312, 1.000000000000000000, 0.9755282581475767101, 0.9755282581475768211 ) ) 
 REPRESENTATION_ITEM ( '' )  );
#32124=CARTESIAN_POINT ( 'NONE',  ( -18.94512977948575738, 13.42499999726881654, -13.76444248337723231 ) ) ;
#32151=CARTESIAN_POINT ( 'NONE',  ( -15.14183272437241889, 18.44999999453764161, -20.84094480462497856 ) ) ;
#32167=CARTESIAN_POINT ( 'NONE',  ( -18.94512977948575738, 15.92499999726881832, -13.76444248337723231 ) ) ;
#32192=CARTESIAN_POINT ( 'NONE',  ( -7.579748464070165821E-14, 10.49999999999999112, -24.50000000000000000 ) ) ;
#32199=CARTESIAN_POINT ( 'NONE',  ( 9.555238894532166682, 16.99999999999998934, 21.84766023402006141 ) ) ;
#32202=CARTESIAN_POINT ( 'NONE',  ( 6.001560367445586717E-15, 3.249999994537631665, 24.50000000000000000 ) ) ;
#32217=( BOUNDED_CURVE ( )  B_SPLINE_CURVE ( 2, ( #14811, #14641, #3997, #28019, #25451, #17734, #25275, #30234, #1748, #6738, #1927, #17220, #22701 ),
 .UNSPECIFIED., .F., .T. ) 
 B_SPLINE_CURVE_WITH_KNOTS ( ( 3, 2, 2, 2, 2, 2, 3 ),
 ( 0.4166666666666666852, 0.4222222222222222210, 0.4333333333333333481, 0.4444444444444444198, 0.4555555555555555469, 0.4666666666666666741, 0.4722222222222222654 ),
 .UNSPECIFIED. ) 
 CURVE ( )  GEOMETRIC_REPRESENTATION_ITEM ( )  RATIONAL_B_SPLINE_CURVE ( ( 0.9755282581475767101, 0.9755282581475768211, 1.000000000000000000, 0.9510565162951535312, 1.000000000000000000, 0.9510565162951535312, 1.000000000000000000, 0.9510565162951535312, 1.000000000000000000, 0.9510565162951535312, 1.000000000000000000, 0.9755282581475765991, 0.9755282581475767101 ) ) 
 REPRESENTATION_ITEM ( '' )  );
#32233=CARTESIAN_POINT ( 'NONE',  ( 24.50000000000000355, 12.09999999999999787, -7.960532557706203605 ) ) ;
#32236=CARTESIAN_POINT ( 'NONE',  ( -14.47279130897151767, 13.32499999726880624, -19.92008829642072598 ) ) ;
#32240=CARTESIAN_POINT ( 'NONE',  ( 11.74590207350062698, 16.99999999999998579, -20.27301895490997197 ) ) ;
#32250=CARTESIAN_POINT ( 'NONE',  ( 8.998893468610761559, 16.99999999999998579, -21.61938333025141290 ) ) ;
#32265=CARTESIAN_POINT ( 'NONE',  ( 24.50000000000000000, 11.90000000000000213, 7.960532557706212486 ) ) ;
#32268=CARTESIAN_POINT ( 'NONE',  ( -14.47279130897151589, 9.324999997268816898, -19.92008829642072598 ) ) ;
#32288=CARTESIAN_POINT ( 'NONE',  ( -14.47279130897151589, 15.32499999726880269, -19.92008829642072598 ) ) ;
#32301=CARTESIAN_POINT ( 'NONE',  ( -6.668400408272875007E-16, 2.249999994537632553, -24.50000000000000355 ) ) ;
#32304=EDGE_CURVE ( 'NONE', #28296, #476, #16408, .T. ) ;
#32317=CARTESIAN_POINT ( 'NONE',  ( 14.47279130897151767, 5.424999997268823648, -19.92008829642072598 ) ) ;
#32332=CARTESIAN_POINT ( 'NONE',  ( 23.41746824999999887, 17.12499999726882649, 0.000000000000000000 ) ) ;
#32340=CARTESIAN_POINT ( 'NONE',  ( -15.14183272437242778, 1.299999999999988054, 20.84094480462497856 ) ) ;
#32349=CYLINDRICAL_SURFACE ( 'NONE', #6195, 24.50000000000000000 ) ;
#32356=CARTESIAN_POINT ( 'NONE',  ( -15.14183272437242067, 10.70000000000001172, -20.84094480462497856 ) ) ;
#32370=DIRECTION ( 'NONE',  ( 0.000000000000000000, -1.000000000000000000, 0.000000000000000000 ) ) ;
#32396=CARTESIAN_POINT ( 'NONE',  ( -7.570916362186210335, 12.59999999999999964, -23.30088464923126779 ) ) ;
#32400=CARTESIAN_POINT ( 'NONE',  ( -18.94512977948576093, 11.82499999726882578, 13.76444248337722698 ) ) ;
#32403=CARTESIAN_POINT ( 'NONE',  ( 17.11581322672471117, 16.99999999999997868, -16.00041235009445018 ) ) ;
#32433=CARTESIAN_POINT ( 'NONE',  ( -18.94512977948575738, 13.42499999726881654, -13.76444248337723231 ) ) ;
#32459=ORIENTED_EDGE ( 'NONE', *, *, #16924, .F. ) ;
#32478=CARTESIAN_POINT ( 'NONE',  ( -14.47279130897151589, 9.824999997268802687, -19.92008829642072598 ) ) ;
#32488=CARTESIAN_POINT ( 'NONE',  ( 19.82091636218621034, 5.799999999999999822, 14.40073868116559730 ) ) ;
#32495=EDGE_CURVE ( 'NONE', #14665, #19251, #6840, .T. ) ;
#32496=CARTESIAN_POINT ( 'NONE',  ( 7.236395654485760609, 15.52499999726880731, -22.27133577429736633 ) ) ;
#32517=VECTOR ( 'NONE', #25715, 1000.000000000000000 ) ;
#32519=CARTESIAN_POINT ( 'NONE',  ( -7.570916362186215665, 9.149999994537639125, 23.30088464923126423 ) ) ;
#32526=CARTESIAN_POINT ( 'NONE',  ( -14.24229347433699289, 16.99999999999998934, 19.84889707891977650 ) ) ;
#32540=AXIS2_PLACEMENT_3D ( 'NONE', #5723, #13274, #2471 ) ;
#32562=CARTESIAN_POINT ( 'NONE',  ( -19.82091636218621034, 12.80000000000000604, -14.40073868116559552 ) ) ;
#32566=CARTESIAN_POINT ( 'NONE',  ( 7.236395654485755280, 10.22499999726880837, 22.27133577429736988 ) ) ;
#32599=CARTESIAN_POINT ( 'NONE',  ( -18.94512977948575738, 11.42499999726881477, -13.76444248337723231 ) ) ;
#32642=CARTESIAN_POINT ( 'NONE',  ( -6.668400408272875007E-16, 0.5000000000000068834, -24.50000000000000355 ) ) ;
#32649=CARTESIAN_POINT ( 'NONE',  ( 23.41746824999999887, 9.124999997268817609, 0.000000000000000000 ) ) ;
#32661=CARTESIAN_POINT ( 'NONE',  ( 15.14183272437242422, 8.049999994537621717, -20.84094480462497856 ) ) ;
#32663=CARTESIAN_POINT ( 'NONE',  ( 7.236395654485760609, 3.024999997268823293, -22.27133577429736633 ) ) ;
#32686=CARTESIAN_POINT ( 'NONE',  ( 24.50000000000000000, 9.749999994537628112, 0.000000000000000000 ) ) ;
#32693=FACE_OUTER_BOUND ( 'NONE', #31713, .T. ) ;
#32708=ORIENTED_EDGE ( 'NONE', *, *, #7884, .T. ) ;
#32729=CARTESIAN_POINT ( 'NONE',  ( 19.82091636218621389, 12.19999999999998863, -14.40073868116559197 ) ) ;
#32733=CARTESIAN_POINT ( 'NONE',  ( 18.94512977948575738, 8.424999997268811214, 13.76444248337723408 ) ) ;
#32737=CARTESIAN_POINT ( 'NONE',  ( 22.63754132413425069, 16.99999999999998934, 6.041913861037119915 ) ) ;
#32767=CARTESIAN_POINT ( 'NONE',  ( -7.236395654485763274, 10.02499999726880198, 22.27133577429736633 ) ) ;
#32791=CARTESIAN_POINT ( 'NONE',  ( -23.41746825000000243, 2.224999997268808816, 7.608796670333725309 ) ) ;
#32795=ORIENTED_EDGE ( 'NONE', *, *, #26764, .F. ) ;
#32812=CARTESIAN_POINT ( 'NONE',  ( -14.47279130897152122, 6.424999997268821872, 19.92008829642072243 ) ) ;
#32816=B_SPLINE_CURVE_WITH_KNOTS ( 'NONE', 3,
 ( #21913, #29955, #21584, #1116, #16437, #19672, #6288, #19012, #3547, #11601, #16764, #3386, #16599, #16271, #29783, #32199, #26889, #22082, #24322, #11115, #14019, #24811, #19508, #6459, #32030, #27391, #795, #13691, #8527, #8693, #956, #13856, #24642, #16933, #32526, #19177, #3880, #14353 ),
 .UNSPECIFIED., .F., .F.,
 ( 4, 2, 2, 2, 2, 2, 2, 2, 2, 2, 2, 2, 2, 2, 2, 2, 2, 2, 4 ),
 ( 0.000000000000000000, 0.001480261321998002991, 0.002960522643996005981, 0.005921045287992017167, 0.008881567931988023148, 0.01036182925398602614, 0.01184209057598402913, 0.01776313586397604283, 0.01924339718597405449, 0.02072365850797205922, 0.02368418115196807908, 0.02664470379596409547, 0.02960522643996011533, 0.03256574908395613172, 0.03404601040595413991, 0.03552627172795214117, 0.04144731701594418782, 0.04440783965994021115, 0.04736836230393623448 ),
 .UNSPECIFIED. ) ;
#32821=EDGE_CURVE ( 'NONE', #6391, #11531, #11773, .T. ) ;
#32825=CARTESIAN_POINT ( 'NONE',  ( 24.50000000000000000, 7.749999994537626336, 0.000000000000000000 ) ) ;
#32827=CARTESIAN_POINT ( 'NONE',  ( -23.41746825000000243, 5.524999997268821517, -7.608796670333730638 ) ) ;
#32850=CARTESIAN_POINT ( 'NONE',  ( 1.577395562988744260E-15, 4.249999994537624559, -25.76082449383753925 ) ) ;
#32858=DIRECTION ( 'NONE',  ( 0.000000000000000000, -1.000000000000000000, 0.000000000000000000 ) ) ;
#32863=CARTESIAN_POINT ( 'NONE',  ( 18.94512977948575738, 4.924999997268808549, 13.76444248337723408 ) ) ;
#32872=ORIENTED_EDGE ( 'NONE', *, *, #24746, .T. ) ;
#32875=CARTESIAN_POINT ( 'NONE',  ( -24.50000000000000000, 3.000000000000002665, -3.000384657911015469E-15 ) ) ;
#32898=CARTESIAN_POINT ( 'NONE',  ( -23.91461052556157441, 16.99999999999998579, -4.889261515958251536 ) ) ;
#32920=CARTESIAN_POINT ( 'NONE',  ( 0.000000000000000000, 16.99999999999998579, -24.50000000000000000 ) ) ;
#32927=FILL_AREA_STYLE ('',( #28144 ) ) ;
#32930=CARTESIAN_POINT ( 'NONE',  ( -18.94512977948576093, 17.82499999726880446, 13.76444248337722698 ) ) ;
#32932=LINE ( 'NONE', #9432, #12377 ) ;
#32955=CARTESIAN_POINT ( 'NONE',  ( 7.236395654485755280, 2.724999997268801266, 22.27133577429736988 ) ) ;
#32962=ORIENTED_EDGE ( 'NONE', *, *, #13074, .F. ) ;
#32971=CARTESIAN_POINT ( 'NONE',  ( 23.41746824999999887, 0.6249999972688102812, 0.000000000000000000 ) ) ;
#32979=ORIENTED_EDGE ( 'NONE', *, *, #26764, .T. ) ;
#32980=CARTESIAN_POINT ( 'NONE',  ( -23.41746825000000598, 6.224999997268799490, 7.608796670333726198 ) ) ;
#32991=CARTESIAN_POINT ( 'NONE',  ( -7.236395654485763274, 4.024999997268824181, 22.27133577429736633 ) ) ;
#32999=ORIENTED_EDGE ( 'NONE', *, *, #5476, .T. ) ;
#33003=ORIENTED_EDGE ( 'NONE', *, *, #5476, .F. ) ;
#33011=FACE_OUTER_BOUND ( 'NONE', #27069, .T. ) ;
#33017=CARTESIAN_POINT ( 'NONE',  ( -24.50000000000000000, 14.74999999453763166, -3.000384657911015469E-15 ) ) ;
#33019=CARTESIAN_POINT ( 'NONE',  ( 15.14183272437242245, 4.049999994537630599, -20.84094480462497856 ) ) ;
#33029=FACE_OUTER_BOUND ( 'NONE', #14580, .T. ) ;
#33034=CARTESIAN_POINT ( 'NONE',  ( 1.507698388325705758E-15, 1.624999997268827823, -24.62258325217400312 ) ) ;
#33041=EDGE_CURVE ( 'NONE', #19228, #14205, #4106, .T. ) ;
#33050=AXIS2_PLACEMENT_3D ( 'NONE', #21129, #31069, #12885 ) ;
#33065=CARTESIAN_POINT ( 'NONE',  ( 24.50000000000000000, 15.99999999999998579, 0.000000000000000000 ) ) ;
#33074=CARTESIAN_POINT ( 'NONE',  ( -3.880418787951142701, 5.198745712990781698, 24.49999999999999645 ) ) ;
#33105=CARTESIAN_POINT ( 'NONE',  ( -23.41746825000000598, 15.72499999726882081, 7.608796670333726198 ) ) ;
#33106=ADVANCED_FACE ( 'NONE', ( #6797 ), #6967, .T. ) ;
#33130=CARTESIAN_POINT ( 'NONE',  ( 18.94512977948576093, 9.324999997268824004, -13.76444248337722875 ) ) ;
#33150=DIRECTION ( 'NONE',  ( 0.000000000000000000, -1.000000000000000000, 0.000000000000000000 ) ) ;
#33158=CARTESIAN_POINT ( 'NONE',  ( 14.47279130897151767, 15.42499999726879878, -19.92008829642072598 ) ) ;
#33171=CARTESIAN_POINT ( 'NONE',  ( -18.94512977948576093, 18.32499999726880446, 13.76444248337722698 ) ) ;
#33173=( GEOMETRIC_REPRESENTATION_CONTEXT ( 3 ) GLOBAL_UNCERTAINTY_ASSIGNED_CONTEXT ( ( #5032 ) ) GLOBAL_UNIT_ASSIGNED_CONTEXT ( ( #17682, #2220, #15109 ) ) REPRESENTATION_CONTEXT ( 'NONE', 'WORKASPACE' ) );
#33196=CARTESIAN_POINT ( 'NONE',  ( 7.570916362186213000, 6.149999994537635573, -23.30088464923126423 ) ) ;
#33204=CARTESIAN_POINT ( 'NONE',  ( 24.50000000000000000, 1.899999999999998135, 7.960532557706212486 ) ) ;
#33210=CARTESIAN_POINT ( 'NONE',  ( 14.47279130897151767, 5.424999997268823648, -19.92008829642072598 ) ) ;
#33231=CARTESIAN_POINT ( 'NONE',  ( -24.50000000000000000, 5.000000000000004441, -3.000384657911015469E-15 ) ) ;
#33246=CARTESIAN_POINT ( 'NONE',  ( 18.94512977948575738, 16.42499999726882010, 13.76444248337723408 ) ) ;
#33252=CARTESIAN_POINT ( 'NONE',  ( -19.35449145663587700, 16.99999999999998934, -14.56863439756531342 ) ) ;
#33270=CYLINDRICAL_SURFACE ( 'NONE', #5556, 24.50000000000000000 ) ;
#33276=FACE_BOUND ( 'NONE', #7867, .T. ) ;
#33281=CARTESIAN_POINT ( 'NONE',  ( 24.50000000000000000, 13.74999999453763166, 0.000000000000000000 ) ) ;
#33286=CARTESIAN_POINT ( 'NONE',  ( 7.236395654485760609, 15.02499999726880731, -22.27133577429736633 ) ) ;
#33311=CARTESIAN_POINT ( 'NONE',  ( -4.523095164977117273E-15, 10.62499999726880517, 24.62258325217400312 ) ) ;
#33329=CARTESIAN_POINT ( 'NONE',  ( 23.95873412499999944, 0.3124999986344190184, 0.000000000000000000 ) ) ;
#33336=CARTESIAN_POINT ( 'NONE',  ( -18.94512977948576093, 14.32499999726880091, 13.76444248337722698 ) ) ;
#33350=CARTESIAN_POINT ( 'NONE',  ( -18.94512977948576093, 3.824999997268818674, 13.76444248337722698 ) ) ;
#33353=EDGE_CURVE ( 'NONE', #27958, #21102, #9356, .T. ) ;
#33375=CARTESIAN_POINT ( 'NONE',  ( 24.50000000000000000, 13.74999999453763166, 0.000000000000000000 ) ) ;
#33388=CARTESIAN_POINT ( 'NONE',  ( 7.236395654485755280, 2.724999997268801266, 22.27133577429736988 ) ) ;
#33397=EDGE_CURVE ( 'NONE', #28001, #16741, #6760, .T. ) ;
#33402=CARTESIAN_POINT ( 'NONE',  ( 24.50000000000000000, 9.900000000000007461, 7.960532557706212486 ) ) ;
#33403=CARTESIAN_POINT ( 'NONE',  ( -15.14183272437242778, 9.049999994537618164, 20.84094480462497856 ) ) ;
#33424=CARTESIAN_POINT ( 'NONE',  ( 7.236395654485755280, 16.22499999726881370, 22.27133577429736988 ) ) ;
#33427=CARTESIAN_POINT ( 'NONE',  ( -24.46341963991828550, 16.99999999999998579, -0.9880410939973442996 ) ) ;
#33435=DIRECTION ( 'NONE',  ( 0.000000000000000000, 1.000000000000000000, 0.000000000000000000 ) ) ;
#33458=CARTESIAN_POINT ( 'NONE',  ( 23.41746825000000243, 14.72499999726881903, -7.608796670333727974 ) ) ;
#33485=CARTESIAN_POINT ( 'NONE',  ( 1.507698388325705758E-15, 5.624999997268818497, -24.62258325217400312 ) ) ;
#33486=VERTEX_POINT ( 'NONE', #22945 ) ;
#33508=VERTEX_POINT ( 'NONE', #23113 ) ;
#33509=CARTESIAN_POINT ( 'NONE',  ( -4.523095164977116484E-15, 14.62499999726882649, 24.62258325217400312 ) ) ;
#33510=CARTESIAN_POINT ( 'NONE',  ( -14.47279130897151767, 7.324999997268822227, -19.92008829642072598 ) ) ;
#33516=UNCERTAINTY_MEASURE_WITH_UNIT (LENGTH_MEASURE( 1.000000000000000082E-05 ), #16877, 'distance_accuracy_value', 'NONE');
#33524=CARTESIAN_POINT ( 'NONE',  ( 23.41746825000000243, 8.524999997268812635, 7.608796670333735079 ) ) ;
#33546=CARTESIAN_POINT ( 'NONE',  ( -19.82091636218621389, 14.94999999453763806, 14.40073868116558842 ) ) ;
#33548=CARTESIAN_POINT ( 'NONE',  ( -24.50000000000000000, 12.74999999453763166, -3.000384657911015469E-15 ) ) ;
#33565=CARTESIAN_POINT ( 'NONE',  ( -14.47279130897152122, 6.424999997268821872, 19.92008829642072243 ) ) ;
#33598=CARTESIAN_POINT ( 'NONE',  ( -14.47279130897152299, 13.92499999726881654, 19.92008829642072243 ) ) ;
#33634=CARTESIAN_POINT ( 'NONE',  ( -4.732186688966233175E-15, 1.500000000000010880, 25.76082449383753925 ) ) ;
#33659=CARTESIAN_POINT ( 'NONE',  ( -18.94512977948575738, 5.924999997268809437, -13.76444248337723231 ) ) ;
#33686=CARTESIAN_POINT ( 'NONE',  ( 14.47279130897151767, 13.42499999726880411, -19.92008829642072598 ) ) ;
#33687=CARTESIAN_POINT ( 'NONE',  ( -18.94512977948575738, 5.424999997268809437, -13.76444248337723231 ) ) ;
#33701=CARTESIAN_POINT ( 'NONE',  ( -4.523095164977116484E-15, 8.124999997268826490, 24.62258325217400312 ) ) ;
#33702=EDGE_CURVE ( 'NONE', #3731, #1393, #1232, .T. ) ;
#33714=AXIS2_PLACEMENT_3D ( 'NONE', #12891, #3108, #18392 ) ;
#33726=CARTESIAN_POINT ( 'NONE',  ( -7.570916362186210335, 14.34999999453762065, -23.30088464923126779 ) ) ;
#33728=CARTESIAN_POINT ( 'NONE',  ( -15.14183272437242600, 11.04999999453761284, 20.84094480462497856 ) ) ;
#33740=SHAPE_REPRESENTATION ( 'connector', ( #1376 ), #33173 ) ;
#33744=CARTESIAN_POINT ( 'NONE',  ( 7.236395654485760609, 11.52499999726880375, -22.27133577429736633 ) ) ;
#33757=CARTESIAN_POINT ( 'NONE',  ( 24.50000000000000000, 10.00000000000000888, 0.000000000000000000 ) ) ;
#33765=CARTESIAN_POINT ( 'NONE',  ( 3.445340210940985210E-14, 5.499999999999997335, 24.50000000000000000 ) ) ;
#33782=CARTESIAN_POINT ( 'NONE',  ( 0.000000000000000000, 16.99999999999998579, 0.000000000000000000 ) ) ;
#33786=CARTESIAN_POINT ( 'NONE',  ( 0.000000000000000000, 16.99999999999998579, 0.000000000000000000 ) ) ;
#33787=CARTESIAN_POINT ( 'NONE',  ( 3.000384657911015469E-15, 16.99999999999998579, 24.50000000000000000 ) ) ;
#33812=CARTESIAN_POINT ( 'NONE',  ( 7.570916362186213000, 6.399999999999988809, -23.30088464923126423 ) ) ;
#33822=FACE_OUTER_BOUND ( 'NONE', #4706, .T. ) ;
#33833=CARTESIAN_POINT ( 'NONE',  ( -23.41746824999999887, 10.02499999726882507, -7.608796670333730638 ) ) ;
#33851=CARTESIAN_POINT ( 'NONE',  ( -23.41746824999999887, 5.624999997268814944, -2.867812753649727150E-15 ) ) ;
#33860=CARTESIAN_POINT ( 'NONE',  ( -7.236395654485757944, 15.72499999726881192, -22.27133577429736988 ) ) ;
#33872=CARTESIAN_POINT ( 'NONE',  ( -18.94512977948575738, 9.424999997268812990, -13.76444248337723231 ) ) ;
#33874=VERTEX_POINT ( 'NONE', #16173 ) ;
#33883=EDGE_LOOP ( 'NONE', ( #30777, #13030, #28724, #3235 ) ) ;
#33898=CARTESIAN_POINT ( 'NONE',  ( -15.14183272437241889, 14.44999999453762207, -20.84094480462497856 ) ) ;
#33914=CARTESIAN_POINT ( 'NONE',  ( 23.41746824999999887, 7.124999997268815832, 0.000000000000000000 ) ) ;
#33947=CARTESIAN_POINT ( 'NONE',  ( 5.749481115774131901, 16.99999999999999289, -22.78789490266839834 ) ) ;
#33950=CARTESIAN_POINT ( 'NONE',  ( 3.000384657911015469E-15, -20.99999999999998934, 24.50000000000000000 ) ) ;
#33973=( NAMED_UNIT ( * ) PLANE_ANGLE_UNIT ( ) SI_UNIT ( $, .RADIAN. ) );
#33976=CARTESIAN_POINT ( 'NONE',  ( -7.570916362186210335, 6.599999999999994316, -23.30088464923126779 ) ) ;
#33978=CARTESIAN_POINT ( 'NONE',  ( -15.14183272437241889, 2.449999994537622960, -20.84094480462497856 ) ) ;
#33985=CARTESIAN_POINT ( 'NONE',  ( 0.000000000000000000, -20.99999999999998934, -26.50000000000000355 ) ) ;
ENDSEC;
END-ISO-10303-21;
